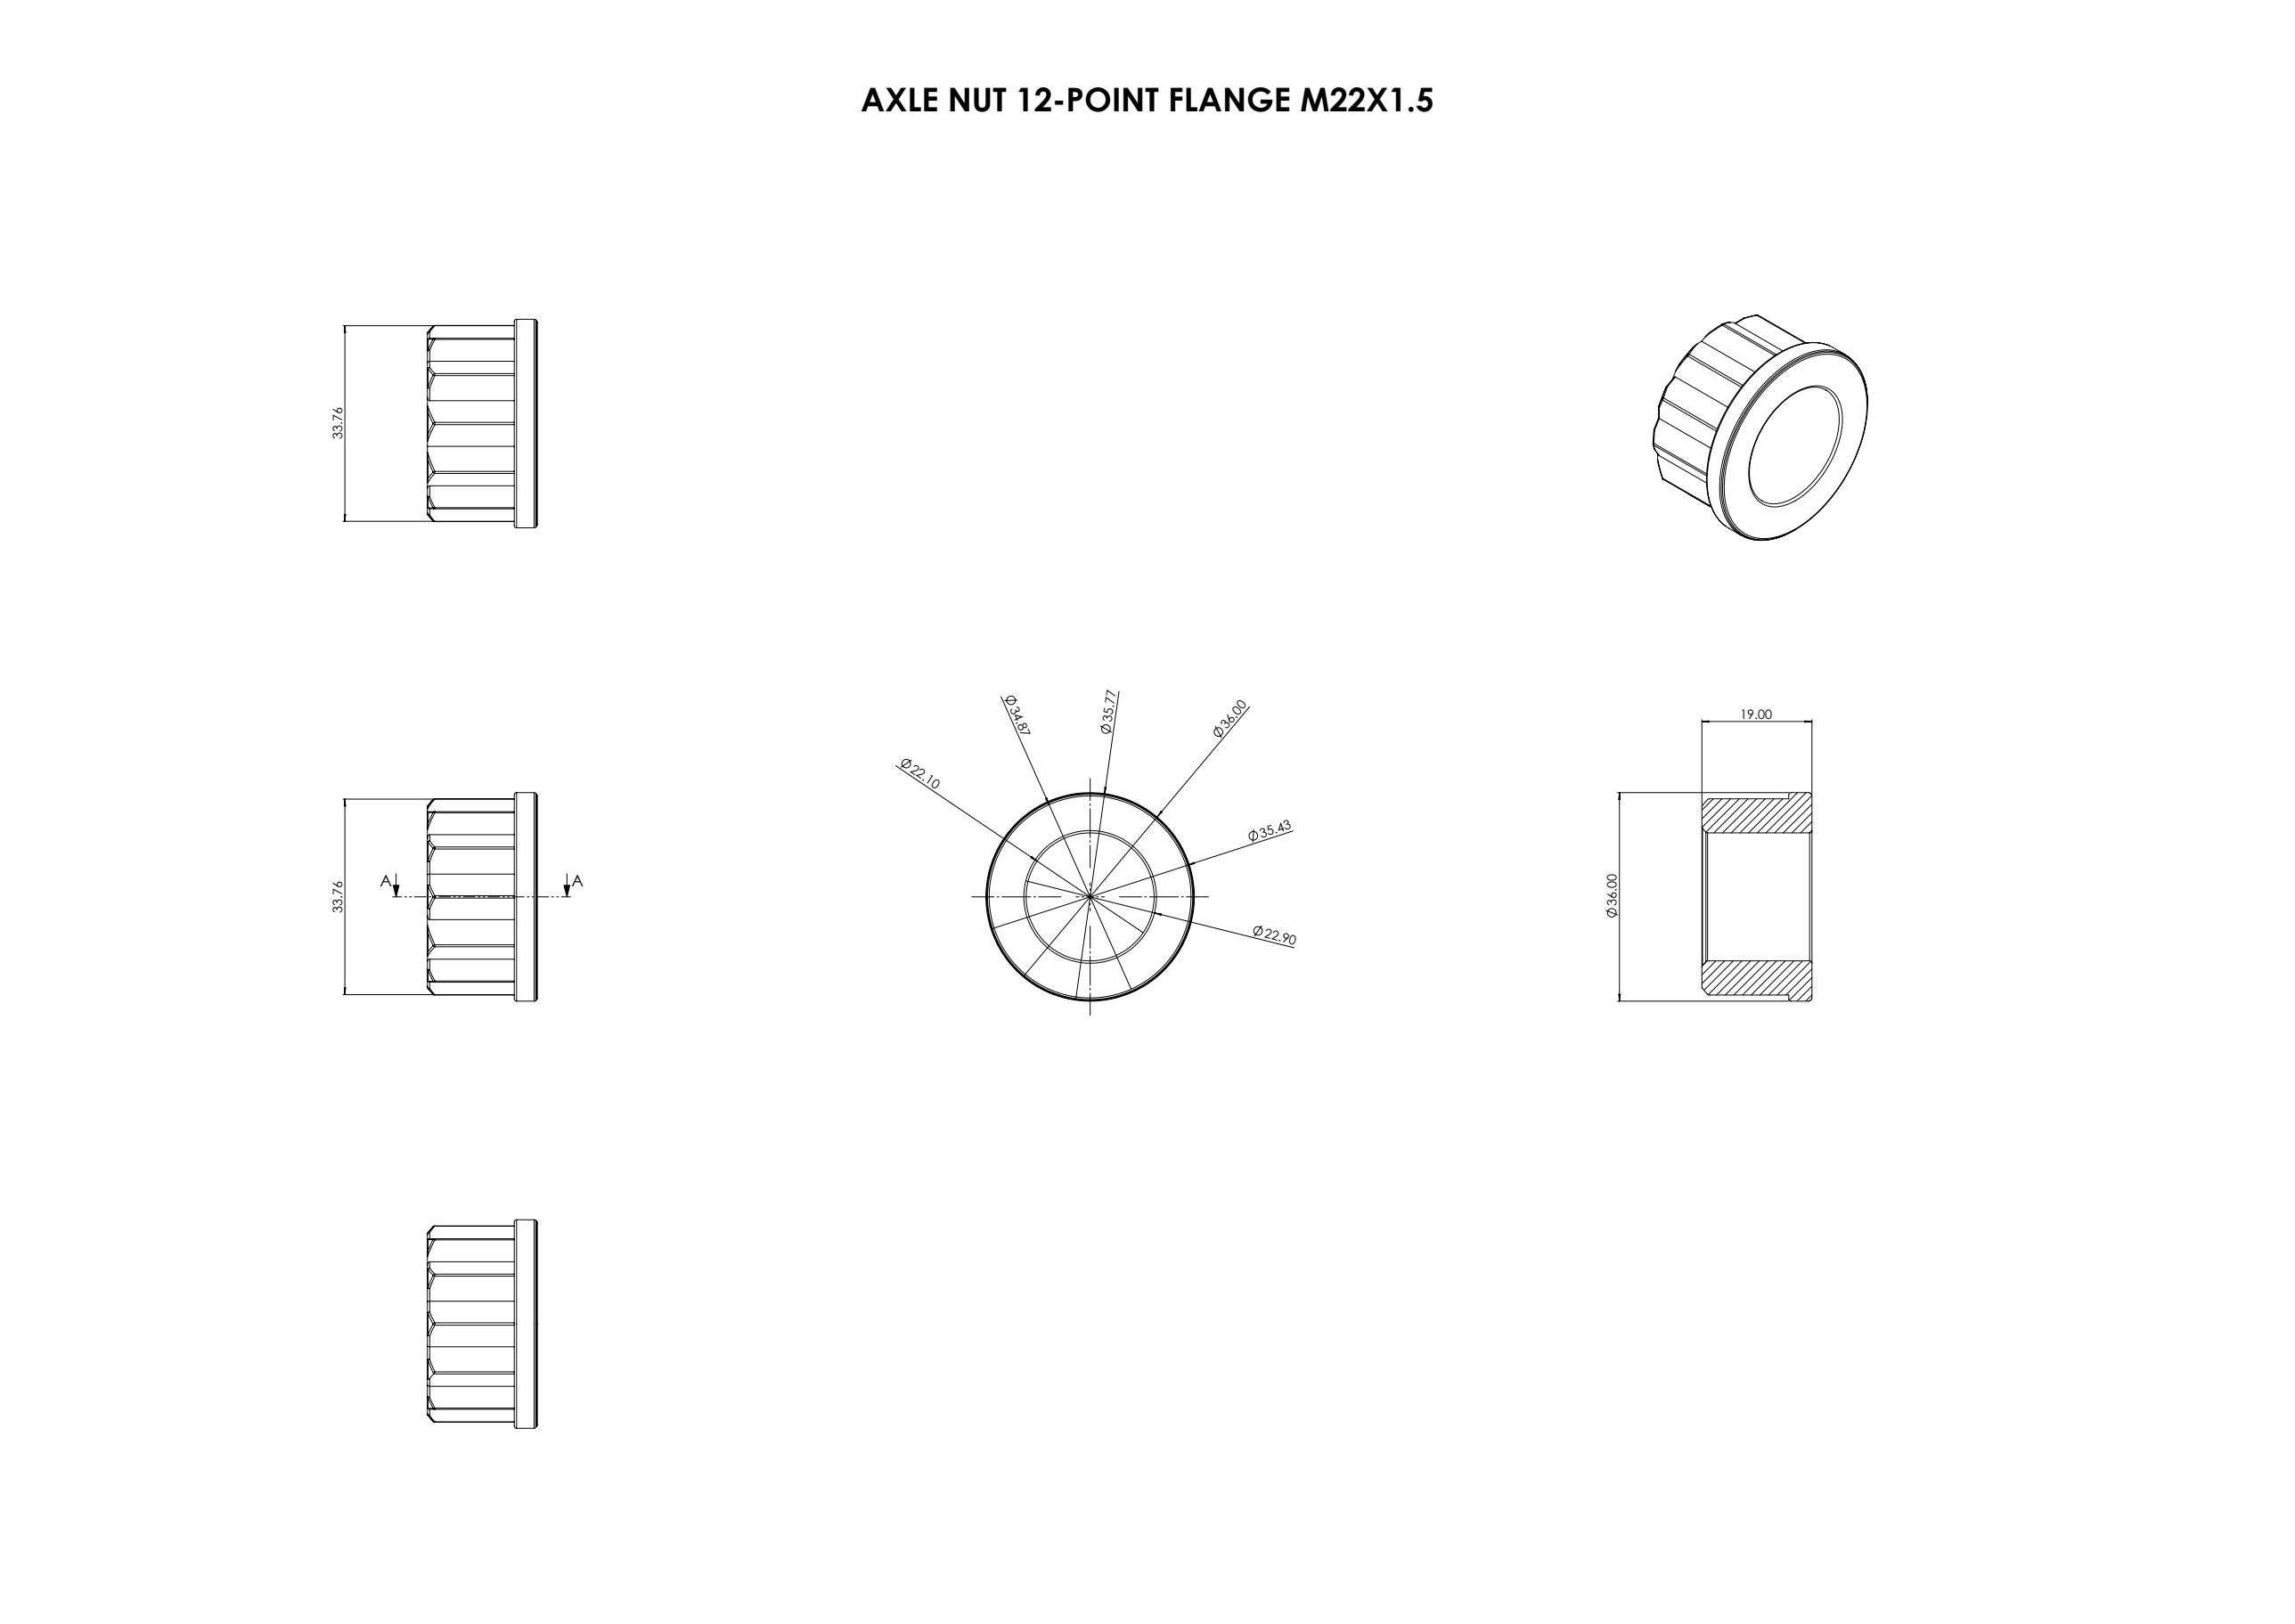
ISO-10303-21;
HEADER;
/* Generated by software containing ST-Developer
 * from STEP Tools, Inc. (www.steptools.com) 
 */

FILE_DESCRIPTION(
/* description */ (''),
/* implementation_level */ '2;1');

FILE_NAME(
/* name */ '03_Axle_Nut_12-Point_Flange_M22x1.5.step',
/* time_stamp */ '2026-10-11T12:57:03-07:00',
/* author */ (''),
/* organization */ (''),
/* preprocessor_version */ 'ST-DEVELOPER v20.2',
/* originating_system */ 'Autodesk Translation Framework v15.15.0.0',
/* authorisation */ '');

FILE_SCHEMA (('AUTOMOTIVE_DESIGN { 1 0 10303 214 3 1 1 }'));
ENDSEC;

DATA;
#10=MECHANICAL_DESIGN_GEOMETRIC_PRESENTATION_REPRESENTATION('',(#258),#90374);
#211=ELLIPSE('',#43033,0.776351396846868,0.4);
#212=ELLIPSE('',#43090,0.415109817788689,0.4);
#213=ELLIPSE('',#43102,0.776351396846869,0.4);
#214=ELLIPSE('',#43130,0.415109817788689,0.4);
#215=ELLIPSE('',#43133,0.41510981778869,0.4);
#216=ELLIPSE('',#43137,0.415109817788689,0.4);
#217=ELLIPSE('',#43157,0.41510981778869,0.4);
#218=ELLIPSE('',#43169,0.415109817788689,0.4);
#219=ELLIPSE('',#43208,0.776351396846868,0.4);
#220=ELLIPSE('',#43220,0.415109817788689,0.4);
#221=ELLIPSE('',#43243,0.776351396846868,0.4);
#224=SHAPE_REPRESENTATION_RELATIONSHIP('SRR','None',#90443,#241);
#241=ADVANCED_BREP_SHAPE_REPRESENTATION('',(#275),#90359);
#258=STYLED_ITEM('',(#90694),#275);
#275=MANIFOLD_SOLID_BREP('Body1',#40347);
#505=SPHERICAL_SURFACE('',#43027,0.4);
#506=SPHERICAL_SURFACE('',#43059,0.4);
#507=SPHERICAL_SURFACE('',#43061,0.4);
#508=SPHERICAL_SURFACE('',#43083,0.4);
#509=SPHERICAL_SURFACE('',#43093,0.4);
#510=SPHERICAL_SURFACE('',#43095,0.4);
#511=SPHERICAL_SURFACE('',#43105,0.4);
#512=SPHERICAL_SURFACE('',#43109,0.4);
#513=SPHERICAL_SURFACE('',#43121,0.4);
#514=SPHERICAL_SURFACE('',#43142,0.4);
#515=SPHERICAL_SURFACE('',#43145,0.4);
#516=SPHERICAL_SURFACE('',#43147,0.4);
#517=SPHERICAL_SURFACE('',#43160,0.4);
#518=SPHERICAL_SURFACE('',#43172,0.399999999999999);
#519=SPHERICAL_SURFACE('',#43181,0.4);
#520=SPHERICAL_SURFACE('',#43183,0.4);
#521=SPHERICAL_SURFACE('',#43185,0.4);
#522=SPHERICAL_SURFACE('',#43187,0.4);
#523=SPHERICAL_SURFACE('',#43189,0.4);
#524=SPHERICAL_SURFACE('',#43202,0.4);
#525=SPHERICAL_SURFACE('',#43210,0.4);
#526=SPHERICAL_SURFACE('',#43225,0.4);
#527=SPHERICAL_SURFACE('',#43228,0.4);
#528=SPHERICAL_SURFACE('',#43231,0.4);
#529=SPHERICAL_SURFACE('',#43237,0.4);
#530=SPHERICAL_SURFACE('',#43244,0.4);
#531=SPHERICAL_SURFACE('',#43258,0.4);
#532=SPHERICAL_SURFACE('',#43261,0.4);
#673=CONICAL_SURFACE('',#43008,17.8,0.785398163397448);
#674=CONICAL_SURFACE('',#43050,11.55,0.83798122500839);
#675=CONICAL_SURFACE('',#43065,16.55,0.840896668643165);
#676=CONICAL_SURFACE('',#43114,16.55,0.840896668643165);
#677=CONICAL_SURFACE('',#43124,16.55,0.840896668643165);
#678=CONICAL_SURFACE('',#43127,16.55,0.840896668643165);
#679=CONICAL_SURFACE('',#43152,16.55,0.840896668643165);
#680=CONICAL_SURFACE('',#43191,16.55,0.840896668643165);
#681=CONICAL_SURFACE('',#43194,16.55,0.840896668643165);
#682=CONICAL_SURFACE('',#43209,16.55,0.840896668643165);
#683=CONICAL_SURFACE('',#43229,16.55,0.840896668643165);
#684=CONICAL_SURFACE('',#43262,16.55,0.840896668643165);
#685=CONICAL_SURFACE('',#43267,16.55,0.840896668643165);
#686=CONICAL_SURFACE('',#43271,16.55,0.840896668643165);
#955=TOROIDAL_SURFACE('',#42999,17.6,0.4);
#956=TOROIDAL_SURFACE('',#43011,17.6,0.4);
#957=TOROIDAL_SURFACE('',#43034,17.4343145750508,0.4);
#958=TOROIDAL_SURFACE('',#43039,11.45,0.4);
#959=TOROIDAL_SURFACE('',#43046,11.45,0.4);
#960=TOROIDAL_SURFACE('',#43067,15.5589388807538,0.4);
#961=TOROIDAL_SURFACE('',#43111,15.5589388807538,0.4);
#962=TOROIDAL_SURFACE('',#43126,15.5589388807538,0.4);
#963=TOROIDAL_SURFACE('',#43131,15.5589388807538,0.4);
#964=TOROIDAL_SURFACE('',#43149,15.5589388807538,0.4);
#965=TOROIDAL_SURFACE('',#43193,15.5589388807538,0.4);
#966=TOROIDAL_SURFACE('',#43196,15.5589388807538,0.4);
#967=TOROIDAL_SURFACE('',#43203,12.0923832909811,0.4);
#968=TOROIDAL_SURFACE('',#43205,15.5589388807538,0.4);
#969=TOROIDAL_SURFACE('',#43221,15.5589388807538,0.4);
#970=TOROIDAL_SURFACE('',#43254,15.5589388807538,0.4);
#971=TOROIDAL_SURFACE('',#43264,15.5589388807538,0.4);
#972=TOROIDAL_SURFACE('',#43268,15.5589388807538,0.4);
#1049=FACE_BOUND('',#5817,.T.);
#1050=FACE_BOUND('',#5825,.T.);
#1051=FACE_BOUND('',#5840,.T.);
#1302=PLANE('',#43014);
#1303=PLANE('',#43032);
#1304=PLANE('',#43037);
#1305=PLANE('',#43063);
#1306=PLANE('',#43070);
#1307=PLANE('',#43097);
#1308=PLANE('',#43099);
#1309=PLANE('',#43116);
#1310=PLANE('',#43123);
#1311=PLANE('',#43134);
#1312=PLANE('',#43148);
#1313=PLANE('',#43190);
#1314=PLANE('',#43197);
#1315=PLANE('',#43198);
#1316=PLANE('',#43199);
#1317=PLANE('',#43207);
#1318=PLANE('',#43215);
#1319=PLANE('',#43230);
#1320=PLANE('',#43236);
#1321=PLANE('',#43242);
#1322=PLANE('',#43249);
#1323=PLANE('',#43263);
#1324=PLANE('',#43266);
#1325=PLANE('',#43270);
#1326=PLANE('',#43272);
#1327=PLANE('',#43273);
#1328=PLANE('',#43274);
#1830=(
BOUNDED_CURVE()
B_SPLINE_CURVE(2,(#77759,#77760,#77761),.UNSPECIFIED.,.F.,.F.)
B_SPLINE_CURVE_WITH_KNOTS((3,3),(0.123046239516649,0.293199132396535),
 .UNSPECIFIED.)
CURVE()
GEOMETRIC_REPRESENTATION_ITEM()
RATIONAL_B_SPLINE_CURVE((1.00286885652603,1.0040332208536,1.00293190037169))
REPRESENTATION_ITEM('')
);
#2083=B_SPLINE_SURFACE_WITH_KNOTS('',3,3,((#77247,#77248,#77249,#77250),
(#77251,#77252,#77253,#77254),(#77255,#77256,#77257,#77258),(#77259,#77260,
#77261,#77262)),.UNSPECIFIED.,.F.,.F.,.F.,(4,4),(4,4),(0.,1.),(0.238859576382585,
0.597949259053295),.UNSPECIFIED.);
#2084=B_SPLINE_SURFACE_WITH_KNOTS('',3,3,((#77282,#77283,#77284,#77285),
(#77286,#77287,#77288,#77289),(#77290,#77291,#77292,#77293),(#77294,#77295,
#77296,#77297)),.UNSPECIFIED.,.F.,.F.,.F.,(4,4),(4,4),(0.,1.),(0.161384884357676,
0.520475215840057),.UNSPECIFIED.);
#2085=B_SPLINE_SURFACE_WITH_KNOTS('',3,3,((#77359,#77360,#77361,#77362),
(#77363,#77364,#77365,#77366),(#77367,#77368,#77369,#77370),(#77371,#77372,
#77373,#77374)),.UNSPECIFIED.,.F.,.F.,.F.,(4,4),(4,4),(0.,1.),(0.,0.231241687907805),
 .UNSPECIFIED.);
#2086=B_SPLINE_SURFACE_WITH_KNOTS('',3,3,((#77406,#77407,#77408,#77409),
(#77410,#77411,#77412,#77413),(#77414,#77415,#77416,#77417),(#77418,#77419,
#77420,#77421)),.UNSPECIFIED.,.F.,.F.,.F.,(4,4),(4,4),(0.,1.),(0.232923065268537,
0.464164679032266),.UNSPECIFIED.);
#2087=B_SPLINE_SURFACE_WITH_KNOTS('',3,3,((#77539,#77540,#77541,#77542),
(#77543,#77544,#77545,#77546),(#77547,#77548,#77549,#77550),(#77551,#77552,
#77553,#77554)),.UNSPECIFIED.,.F.,.F.,.F.,(4,4),(4,4),(0.,1.),(0.,0.23124168790661),
 .UNSPECIFIED.);
#2088=B_SPLINE_SURFACE_WITH_KNOTS('',3,3,((#77572,#77573,#77574,#77575),
(#77576,#77577,#77578,#77579),(#77580,#77581,#77582,#77583),(#77584,#77585,
#77586,#77587)),.UNSPECIFIED.,.F.,.F.,.F.,(4,4),(4,4),(0.,1.),(0.,0.2312416879078),
 .UNSPECIFIED.);
#2089=B_SPLINE_SURFACE_WITH_KNOTS('',3,3,((#77617,#77618,#77619,#77620),
(#77621,#77622,#77623,#77624),(#77625,#77626,#77627,#77628),(#77629,#77630,
#77631,#77632)),.UNSPECIFIED.,.F.,.F.,.F.,(4,4),(4,4),(0.,1.),(0.,0.231241687907749),
 .UNSPECIFIED.);
#2090=B_SPLINE_SURFACE_WITH_KNOTS('',3,3,((#77664,#77665,#77666,#77667),
(#77668,#77669,#77670,#77671),(#77672,#77673,#77674,#77675),(#77676,#77677,
#77678,#77679)),.UNSPECIFIED.,.F.,.F.,.F.,(4,4),(4,4),(0.,1.),(0.,0.231241350797188),
 .UNSPECIFIED.);
#2091=B_SPLINE_SURFACE_WITH_KNOTS('',3,3,((#77725,#77726,#77727,#77728),
(#77729,#77730,#77731,#77732),(#77733,#77734,#77735,#77736),(#77737,#77738,
#77739,#77740)),.UNSPECIFIED.,.F.,.F.,.F.,(4,4),(4,4),(0.,1.),(0.,0.252215655062094),
 .UNSPECIFIED.);
#2092=B_SPLINE_SURFACE_WITH_KNOTS('',3,3,((#77807,#77808,#77809,#77810),
(#77811,#77812,#77813,#77814),(#77815,#77816,#77817,#77818),(#77819,#77820,
#77821,#77822)),.UNSPECIFIED.,.F.,.F.,.F.,(4,4),(4,4),(0.,1.),(0.,0.231241687907802),
 .UNSPECIFIED.);
#2093=B_SPLINE_SURFACE_WITH_KNOTS('',3,3,((#77857,#77858,#77859,#77860),
(#77861,#77862,#77863,#77864),(#77865,#77866,#77867,#77868),(#77869,#77870,
#77871,#77872)),.UNSPECIFIED.,.F.,.F.,.F.,(4,4),(4,4),(0.,1.),(0.,0.231241586165377),
 .UNSPECIFIED.);
#2094=B_SPLINE_SURFACE_WITH_KNOTS('',3,3,((#77898,#77899,#77900,#77901),
(#77902,#77903,#77904,#77905),(#77906,#77907,#77908,#77909),(#77910,#77911,
#77912,#77913)),.UNSPECIFIED.,.F.,.F.,.F.,(4,4),(4,4),(0.,1.),(0.,0.23124114363781),
 .UNSPECIFIED.);
#2095=B_SPLINE_SURFACE_WITH_KNOTS('',3,3,((#77925,#77926,#77927,#77928),
(#77929,#77930,#77931,#77932),(#77933,#77934,#77935,#77936),(#77937,#77938,
#77939,#77940)),.UNSPECIFIED.,.F.,.F.,.F.,(4,4),(4,4),(0.,1.),(0.228586915697378,
0.459828059335187),.UNSPECIFIED.);
#2096=B_SPLINE_SURFACE_WITH_KNOTS('',3,3,((#77970,#77971,#77972,#77973),
(#77974,#77975,#77976,#77977),(#77978,#77979,#77980,#77981),(#77982,#77983,
#77984,#77985)),.UNSPECIFIED.,.F.,.F.,.F.,(4,4),(4,4),(0.,1.),(0.,0.231241350797186),
 .UNSPECIFIED.);
#2097=B_SPLINE_SURFACE_WITH_KNOTS('',3,3,((#77997,#77998,#77999,#78000),
(#78001,#78002,#78003,#78004),(#78005,#78006,#78007,#78008),(#78009,#78010,
#78011,#78012)),.UNSPECIFIED.,.F.,.F.,.F.,(4,4),(4,4),(0.,1.),(0.215800706400213,
0.447042292565588),.UNSPECIFIED.);
#2098=B_SPLINE_SURFACE_WITH_KNOTS('',3,3,((#78076,#78077,#78078,#78079),
(#78080,#78081,#78082,#78083),(#78084,#78085,#78086,#78087),(#78088,#78089,
#78090,#78091)),.UNSPECIFIED.,.F.,.F.,.F.,(4,4),(4,4),(0.,1.),(0.228585906851782,
0.459827831361922),.UNSPECIFIED.);
#2099=B_SPLINE_SURFACE_WITH_KNOTS('',3,3,((#78098,#78099,#78100,#78101),
(#78102,#78103,#78104,#78105),(#78106,#78107,#78108,#78109),(#78110,#78111,
#78112,#78113)),.UNSPECIFIED.,.F.,.F.,.F.,(4,4),(4,4),(0.,1.),(0.289233280455309,
0.520475100360999),.UNSPECIFIED.);
#2100=B_SPLINE_SURFACE_WITH_KNOTS('',3,3,((#78157,#78158,#78159,#78160),
(#78161,#78162,#78163,#78164),(#78165,#78166,#78167,#78168),(#78169,#78170,
#78171,#78172)),.UNSPECIFIED.,.F.,.F.,.F.,(4,4),(4,4),(0.,1.),(0.228585906851781,
0.587676103485633),.UNSPECIFIED.);
#2101=B_SPLINE_SURFACE_WITH_KNOTS('',3,3,((#78184,#78185,#78186,#78187),
(#78188,#78189,#78190,#78191),(#78192,#78193,#78194,#78195),(#78196,#78197,
#78198,#78199)),.UNSPECIFIED.,.F.,.F.,.F.,(4,4),(4,4),(0.,1.),(0.157372832782455,
0.516463029416307),.UNSPECIFIED.);
#2102=B_SPLINE_SURFACE_WITH_KNOTS('',3,3,((#78233,#78234,#78235,#78236),
(#78237,#78238,#78239,#78240),(#78241,#78242,#78243,#78244),(#78245,#78246,
#78247,#78248)),.UNSPECIFIED.,.F.,.F.,.F.,(4,4),(4,4),(0.,1.),(0.238859576382585,
0.597949259053296),.UNSPECIFIED.);
#2103=B_SPLINE_SURFACE_WITH_KNOTS('',3,3,((#78260,#78261,#78262,#78263),
(#78264,#78265,#78266,#78267),(#78268,#78269,#78270,#78271),(#78272,#78273,
#78274,#78275)),.UNSPECIFIED.,.F.,.F.,.F.,(4,4),(4,4),(0.,1.),(0.14489400298759,
0.503986701734181),.UNSPECIFIED.);
#2104=B_SPLINE_SURFACE_WITH_KNOTS('',3,3,((#78308,#78309,#78310,#78311),
(#78312,#78313,#78314,#78315),(#78316,#78317,#78318,#78319),(#78320,#78321,
#78322,#78323)),.UNSPECIFIED.,.F.,.F.,.F.,(4,4),(4,4),(0.,1.),(0.232923065268538,
0.464164679032267),.UNSPECIFIED.);
#2105=B_SPLINE_SURFACE_WITH_KNOTS('',3,3,((#78330,#78331,#78332,#78333),
(#78334,#78335,#78336,#78337),(#78338,#78339,#78340,#78341),(#78342,#78343,
#78344,#78345)),.UNSPECIFIED.,.F.,.F.,.F.,(4,4),(4,4),(0.,1.),(0.27134084970268,
0.502582702411899),.UNSPECIFIED.);
#3406=FACE_OUTER_BOUND('',#5812,.T.);
#3407=FACE_OUTER_BOUND('',#5813,.T.);
#3408=FACE_OUTER_BOUND('',#5814,.T.);
#3409=FACE_OUTER_BOUND('',#5815,.T.);
#3410=FACE_OUTER_BOUND('',#5816,.T.);
#3411=FACE_OUTER_BOUND('',#5818,.T.);
#3412=FACE_OUTER_BOUND('',#5819,.T.);
#3413=FACE_OUTER_BOUND('',#5820,.T.);
#3414=FACE_OUTER_BOUND('',#5821,.T.);
#3415=FACE_OUTER_BOUND('',#5822,.T.);
#3416=FACE_OUTER_BOUND('',#5823,.T.);
#3417=FACE_OUTER_BOUND('',#5824,.T.);
#3418=FACE_OUTER_BOUND('',#5826,.T.);
#3419=FACE_OUTER_BOUND('',#5827,.T.);
#3420=FACE_OUTER_BOUND('',#5828,.T.);
#3421=FACE_OUTER_BOUND('',#5829,.T.);
#3422=FACE_OUTER_BOUND('',#5830,.T.);
#3423=FACE_OUTER_BOUND('',#5831,.T.);
#3424=FACE_OUTER_BOUND('',#5832,.T.);
#3425=FACE_OUTER_BOUND('',#5833,.T.);
#3426=FACE_OUTER_BOUND('',#5834,.T.);
#3427=FACE_OUTER_BOUND('',#5835,.T.);
#3428=FACE_OUTER_BOUND('',#5836,.T.);
#3429=FACE_OUTER_BOUND('',#5837,.T.);
#3430=FACE_OUTER_BOUND('',#5838,.T.);
#3431=FACE_OUTER_BOUND('',#5839,.T.);
#3432=FACE_OUTER_BOUND('',#5841,.T.);
#3433=FACE_OUTER_BOUND('',#5842,.T.);
#3434=FACE_OUTER_BOUND('',#5843,.T.);
#3435=FACE_OUTER_BOUND('',#5844,.T.);
#3436=FACE_OUTER_BOUND('',#5845,.T.);
#3437=FACE_OUTER_BOUND('',#5846,.T.);
#3438=FACE_OUTER_BOUND('',#5847,.T.);
#3439=FACE_OUTER_BOUND('',#5848,.T.);
#3440=FACE_OUTER_BOUND('',#5849,.T.);
#3441=FACE_OUTER_BOUND('',#5850,.T.);
#3442=FACE_OUTER_BOUND('',#5851,.T.);
#3443=FACE_OUTER_BOUND('',#5852,.T.);
#3444=FACE_OUTER_BOUND('',#5853,.T.);
#3445=FACE_OUTER_BOUND('',#5854,.T.);
#3446=FACE_OUTER_BOUND('',#5855,.T.);
#3447=FACE_OUTER_BOUND('',#5856,.T.);
#3448=FACE_OUTER_BOUND('',#5857,.T.);
#3449=FACE_OUTER_BOUND('',#5858,.T.);
#3450=FACE_OUTER_BOUND('',#5859,.T.);
#3451=FACE_OUTER_BOUND('',#5860,.T.);
#3452=FACE_OUTER_BOUND('',#5861,.T.);
#3453=FACE_OUTER_BOUND('',#5862,.T.);
#3454=FACE_OUTER_BOUND('',#5863,.T.);
#3455=FACE_OUTER_BOUND('',#5864,.T.);
#3456=FACE_OUTER_BOUND('',#5865,.T.);
#3457=FACE_OUTER_BOUND('',#5866,.T.);
#3458=FACE_OUTER_BOUND('',#5867,.T.);
#3459=FACE_OUTER_BOUND('',#5868,.T.);
#3460=FACE_OUTER_BOUND('',#5869,.T.);
#3461=FACE_OUTER_BOUND('',#5870,.T.);
#3462=FACE_OUTER_BOUND('',#5871,.T.);
#3463=FACE_OUTER_BOUND('',#5872,.T.);
#3464=FACE_OUTER_BOUND('',#5873,.T.);
#3465=FACE_OUTER_BOUND('',#5874,.T.);
#3466=FACE_OUTER_BOUND('',#5875,.T.);
#3467=FACE_OUTER_BOUND('',#5876,.T.);
#3468=FACE_OUTER_BOUND('',#5877,.T.);
#3469=FACE_OUTER_BOUND('',#5878,.T.);
#3470=FACE_OUTER_BOUND('',#5879,.T.);
#3471=FACE_OUTER_BOUND('',#5880,.T.);
#3472=FACE_OUTER_BOUND('',#5881,.T.);
#3473=FACE_OUTER_BOUND('',#5882,.T.);
#3474=FACE_OUTER_BOUND('',#5883,.T.);
#3475=FACE_OUTER_BOUND('',#5884,.T.);
#3476=FACE_OUTER_BOUND('',#5885,.T.);
#3477=FACE_OUTER_BOUND('',#5886,.T.);
#3478=FACE_OUTER_BOUND('',#5887,.T.);
#3479=FACE_OUTER_BOUND('',#5888,.T.);
#3480=FACE_OUTER_BOUND('',#5889,.T.);
#3481=FACE_OUTER_BOUND('',#5890,.T.);
#3482=FACE_OUTER_BOUND('',#5891,.T.);
#3483=FACE_OUTER_BOUND('',#5892,.T.);
#3484=FACE_OUTER_BOUND('',#5893,.T.);
#3485=FACE_OUTER_BOUND('',#5894,.T.);
#3486=FACE_OUTER_BOUND('',#5895,.T.);
#3487=FACE_OUTER_BOUND('',#5896,.T.);
#3488=FACE_OUTER_BOUND('',#5897,.T.);
#3489=FACE_OUTER_BOUND('',#5898,.T.);
#3490=FACE_OUTER_BOUND('',#5899,.T.);
#3491=FACE_OUTER_BOUND('',#5900,.T.);
#3492=FACE_OUTER_BOUND('',#5901,.T.);
#3493=FACE_OUTER_BOUND('',#5902,.T.);
#3494=FACE_OUTER_BOUND('',#5903,.T.);
#3495=FACE_OUTER_BOUND('',#5904,.T.);
#3496=FACE_OUTER_BOUND('',#5905,.T.);
#3497=FACE_OUTER_BOUND('',#5906,.T.);
#3498=FACE_OUTER_BOUND('',#5907,.T.);
#3499=FACE_OUTER_BOUND('',#5908,.T.);
#3500=FACE_OUTER_BOUND('',#5909,.T.);
#3501=FACE_OUTER_BOUND('',#5910,.T.);
#3502=FACE_OUTER_BOUND('',#5911,.T.);
#3503=FACE_OUTER_BOUND('',#5912,.T.);
#3504=FACE_OUTER_BOUND('',#5913,.T.);
#3505=FACE_OUTER_BOUND('',#5914,.T.);
#3506=FACE_OUTER_BOUND('',#5915,.T.);
#3507=FACE_OUTER_BOUND('',#5916,.T.);
#3508=FACE_OUTER_BOUND('',#5917,.T.);
#3509=FACE_OUTER_BOUND('',#5918,.T.);
#3510=FACE_OUTER_BOUND('',#5919,.T.);
#3511=FACE_OUTER_BOUND('',#5920,.T.);
#3512=FACE_OUTER_BOUND('',#5921,.T.);
#3513=FACE_OUTER_BOUND('',#5922,.T.);
#3514=FACE_OUTER_BOUND('',#5923,.T.);
#3515=FACE_OUTER_BOUND('',#5924,.T.);
#3516=FACE_OUTER_BOUND('',#5925,.T.);
#3517=FACE_OUTER_BOUND('',#5926,.T.);
#3518=FACE_OUTER_BOUND('',#5927,.T.);
#3519=FACE_OUTER_BOUND('',#5928,.T.);
#3520=FACE_OUTER_BOUND('',#5929,.T.);
#3521=FACE_OUTER_BOUND('',#5930,.T.);
#3522=FACE_OUTER_BOUND('',#5931,.T.);
#3523=FACE_OUTER_BOUND('',#5932,.T.);
#3524=FACE_OUTER_BOUND('',#5933,.T.);
#3525=FACE_OUTER_BOUND('',#5934,.T.);
#3526=FACE_OUTER_BOUND('',#5935,.T.);
#3527=FACE_OUTER_BOUND('',#5936,.T.);
#3528=FACE_OUTER_BOUND('',#5937,.T.);
#3529=FACE_OUTER_BOUND('',#5938,.T.);
#3530=FACE_OUTER_BOUND('',#5939,.T.);
#3531=FACE_OUTER_BOUND('',#5940,.T.);
#3532=FACE_OUTER_BOUND('',#5941,.T.);
#3533=FACE_OUTER_BOUND('',#5942,.T.);
#3534=FACE_OUTER_BOUND('',#5943,.T.);
#3535=FACE_OUTER_BOUND('',#5944,.T.);
#3536=FACE_OUTER_BOUND('',#5945,.T.);
#3537=FACE_OUTER_BOUND('',#5946,.T.);
#3538=FACE_OUTER_BOUND('',#5947,.T.);
#3539=FACE_OUTER_BOUND('',#5948,.T.);
#3540=FACE_OUTER_BOUND('',#5949,.T.);
#3541=FACE_OUTER_BOUND('',#5950,.T.);
#3542=FACE_OUTER_BOUND('',#5951,.T.);
#3543=FACE_OUTER_BOUND('',#5952,.T.);
#3544=FACE_OUTER_BOUND('',#5953,.T.);
#3545=FACE_OUTER_BOUND('',#5954,.T.);
#3546=FACE_OUTER_BOUND('',#5955,.T.);
#3547=FACE_OUTER_BOUND('',#5956,.T.);
#5812=EDGE_LOOP('',(#31161,#31162,#31163,#31164,#31165,#31166));
#5813=EDGE_LOOP('',(#31167,#31168,#31169,#31170,#31171,#31172));
#5814=EDGE_LOOP('',(#31173,#31174,#31175,#31176,#31177,#31178));
#5815=EDGE_LOOP('',(#31179,#31180,#31181,#31182,#31183));
#5816=EDGE_LOOP('',(#31184));
#5817=EDGE_LOOP('',(#31185,#31186,#31187,#31188,#31189,#31190,#31191,#31192,
#31193,#31194,#31195,#31196,#31197,#31198,#31199,#31200,#31201,#31202,#31203,
#31204,#31205,#31206,#31207,#31208,#31209,#31210,#31211,#31212,#31213,#31214,
#31215,#31216,#31217,#31218,#31219,#31220));
#5818=EDGE_LOOP('',(#31221,#31222,#31223));
#5819=EDGE_LOOP('',(#31224,#31225,#31226,#31227));
#5820=EDGE_LOOP('',(#31228,#31229,#31230,#31231,#31232,#31233));
#5821=EDGE_LOOP('',(#31234,#31235,#31236,#31237,#31238));
#5822=EDGE_LOOP('',(#31239,#31240,#31241,#31242,#31243));
#5823=EDGE_LOOP('',(#31244,#31245,#31246,#31247,#31248));
#5824=EDGE_LOOP('',(#31249));
#5825=EDGE_LOOP('',(#31250));
#5826=EDGE_LOOP('',(#31251,#31252,#31253,#31254,#31255));
#5827=EDGE_LOOP('',(#31256,#31257,#31258,#31259,#31260,#31261));
#5828=EDGE_LOOP('',(#31262,#31263,#31264,#31265,#31266,#31267));
#5829=EDGE_LOOP('',(#31268,#31269,#31270,#31271,#31272,#31273));
#5830=EDGE_LOOP('',(#31274,#31275,#31276,#31277));
#5831=EDGE_LOOP('',(#31278,#31279,#31280,#31281));
#5832=EDGE_LOOP('',(#31282,#31283,#31284,#31285));
#5833=EDGE_LOOP('',(#31286,#31287,#31288));
#5834=EDGE_LOOP('',(#31289,#31290,#31291));
#5835=EDGE_LOOP('',(#31292,#31293,#31294,#31295,#31296));
#5836=EDGE_LOOP('',(#31297,#31298,#31299,#31300));
#5837=EDGE_LOOP('',(#31301,#31302,#31303));
#5838=EDGE_LOOP('',(#31304,#31305,#31306,#31307));
#5839=EDGE_LOOP('',(#31308,#31309,#31310,#31311,#31312,#31313,#31314,#31315,
#31316,#31317,#31318,#31319,#31320,#31321,#31322,#31323,#31324,#31325,#31326,
#31327,#31328,#31329,#31330,#31331,#31332,#31333,#31334,#31335,#31336,#31337,
#31338,#31339,#31340,#31341,#31342,#31343,#31344,#31345,#31346,#31347,#31348,
#31349));
#5840=EDGE_LOOP('',(#31350));
#5841=EDGE_LOOP('',(#31351,#31352,#31353));
#5842=EDGE_LOOP('',(#31354,#31355,#31356,#31357));
#5843=EDGE_LOOP('',(#31358,#31359,#31360,#31361));
#5844=EDGE_LOOP('',(#31362,#31363,#31364,#31365));
#5845=EDGE_LOOP('',(#31366,#31367,#31368));
#5846=EDGE_LOOP('',(#31369,#31370,#31371));
#5847=EDGE_LOOP('',(#31372,#31373,#31374,#31375,#31376));
#5848=EDGE_LOOP('',(#31377,#31378,#31379,#31380));
#5849=EDGE_LOOP('',(#31381,#31382,#31383,#31384,#31385));
#5850=EDGE_LOOP('',(#31386,#31387,#31388,#31389));
#5851=EDGE_LOOP('',(#31390,#31391,#31392,#31393));
#5852=EDGE_LOOP('',(#31394,#31395,#31396));
#5853=EDGE_LOOP('',(#31397,#31398,#31399,#31400));
#5854=EDGE_LOOP('',(#31401,#31402,#31403));
#5855=EDGE_LOOP('',(#31404,#31405,#31406,#31407));
#5856=EDGE_LOOP('',(#31408,#31409,#31410));
#5857=EDGE_LOOP('',(#31411,#31412,#31413,#31414));
#5858=EDGE_LOOP('',(#31415,#31416,#31417,#31418,#31419));
#5859=EDGE_LOOP('',(#31420,#31421,#31422,#31423,#31424));
#5860=EDGE_LOOP('',(#31425,#31426,#31427,#31428));
#5861=EDGE_LOOP('',(#31429,#31430,#31431,#31432));
#5862=EDGE_LOOP('',(#31433,#31434,#31435));
#5863=EDGE_LOOP('',(#31436,#31437,#31438,#31439,#31440));
#5864=EDGE_LOOP('',(#31441,#31442,#31443,#31444,#31445));
#5865=EDGE_LOOP('',(#31446,#31447,#31448,#31449));
#5866=EDGE_LOOP('',(#31450,#31451,#31452));
#5867=EDGE_LOOP('',(#31453,#31454,#31455,#31456));
#5868=EDGE_LOOP('',(#31457,#31458,#31459,#31460));
#5869=EDGE_LOOP('',(#31461,#31462,#31463,#31464,#31465));
#5870=EDGE_LOOP('',(#31466,#31467,#31468,#31469,#31470));
#5871=EDGE_LOOP('',(#31471,#31472,#31473,#31474));
#5872=EDGE_LOOP('',(#31475,#31476,#31477,#31478));
#5873=EDGE_LOOP('',(#31479,#31480,#31481,#31482));
#5874=EDGE_LOOP('',(#31483,#31484,#31485));
#5875=EDGE_LOOP('',(#31486,#31487,#31488));
#5876=EDGE_LOOP('',(#31489,#31490,#31491));
#5877=EDGE_LOOP('',(#31492,#31493,#31494,#31495,#31496));
#5878=EDGE_LOOP('',(#31497,#31498,#31499,#31500));
#5879=EDGE_LOOP('',(#31501,#31502,#31503));
#5880=EDGE_LOOP('',(#31504,#31505,#31506,#31507));
#5881=EDGE_LOOP('',(#31508,#31509,#31510,#31511));
#5882=EDGE_LOOP('',(#31512,#31513,#31514,#31515));
#5883=EDGE_LOOP('',(#31516,#31517,#31518,#31519));
#5884=EDGE_LOOP('',(#31520,#31521,#31522));
#5885=EDGE_LOOP('',(#31523,#31524,#31525,#31526));
#5886=EDGE_LOOP('',(#31527,#31528,#31529,#31530));
#5887=EDGE_LOOP('',(#31531,#31532,#31533,#31534));
#5888=EDGE_LOOP('',(#31535,#31536,#31537,#31538));
#5889=EDGE_LOOP('',(#31539,#31540,#31541,#31542));
#5890=EDGE_LOOP('',(#31543,#31544,#31545));
#5891=EDGE_LOOP('',(#31546,#31547,#31548,#31549));
#5892=EDGE_LOOP('',(#31550,#31551,#31552,#31553));
#5893=EDGE_LOOP('',(#31554,#31555,#31556,#31557));
#5894=EDGE_LOOP('',(#31558,#31559,#31560,#31561));
#5895=EDGE_LOOP('',(#31562,#31563,#31564));
#5896=EDGE_LOOP('',(#31565,#31566,#31567));
#5897=EDGE_LOOP('',(#31568,#31569,#31570));
#5898=EDGE_LOOP('',(#31571,#31572,#31573));
#5899=EDGE_LOOP('',(#31574,#31575,#31576));
#5900=EDGE_LOOP('',(#31577,#31578,#31579,#31580,#31581));
#5901=EDGE_LOOP('',(#31582,#31583,#31584));
#5902=EDGE_LOOP('',(#31585,#31586,#31587,#31588));
#5903=EDGE_LOOP('',(#31589,#31590,#31591));
#5904=EDGE_LOOP('',(#31592,#31593,#31594,#31595));
#5905=EDGE_LOOP('',(#31596,#31597,#31598,#31599,#31600));
#5906=EDGE_LOOP('',(#31601,#31602,#31603,#31604,#31605));
#5907=EDGE_LOOP('',(#31606,#31607,#31608,#31609,#31610));
#5908=EDGE_LOOP('',(#31611,#31612,#31613,#31614));
#5909=EDGE_LOOP('',(#31615,#31616,#31617));
#5910=EDGE_LOOP('',(#31618,#31619,#31620,#31621,#31622));
#5911=EDGE_LOOP('',(#31623,#31624,#31625,#31626));
#5912=EDGE_LOOP('',(#31627,#31628,#31629,#31630,#31631,#31632));
#5913=EDGE_LOOP('',(#31633,#31634,#31635));
#5914=EDGE_LOOP('',(#31636,#31637,#31638));
#5915=EDGE_LOOP('',(#31639,#31640,#31641,#31642));
#5916=EDGE_LOOP('',(#31643,#31644,#31645,#31646,#31647));
#5917=EDGE_LOOP('',(#31648,#31649,#31650,#31651));
#5918=EDGE_LOOP('',(#31652,#31653,#31654,#31655));
#5919=EDGE_LOOP('',(#31656,#31657,#31658,#31659));
#5920=EDGE_LOOP('',(#31660,#31661,#31662,#31663));
#5921=EDGE_LOOP('',(#31664,#31665,#31666));
#5922=EDGE_LOOP('',(#31667,#31668,#31669,#31670));
#5923=EDGE_LOOP('',(#31671,#31672,#31673));
#5924=EDGE_LOOP('',(#31674,#31675,#31676));
#5925=EDGE_LOOP('',(#31677,#31678,#31679,#31680,#31681));
#5926=EDGE_LOOP('',(#31682,#31683,#31684));
#5927=EDGE_LOOP('',(#31685,#31686,#31687,#31688));
#5928=EDGE_LOOP('',(#31689,#31690,#31691,#31692,#31693));
#5929=EDGE_LOOP('',(#31694,#31695,#31696,#31697,#31698));
#5930=EDGE_LOOP('',(#31699,#31700,#31701,#31702,#31703));
#5931=EDGE_LOOP('',(#31704,#31705,#31706));
#5932=EDGE_LOOP('',(#31707,#31708,#31709,#31710));
#5933=EDGE_LOOP('',(#31711,#31712,#31713,#31714,#31715,#31716));
#5934=EDGE_LOOP('',(#31717,#31718,#31719,#31720,#31721));
#5935=EDGE_LOOP('',(#31722,#31723,#31724,#31725,#31726));
#5936=EDGE_LOOP('',(#31727,#31728,#31729));
#5937=EDGE_LOOP('',(#31730,#31731,#31732,#31733));
#5938=EDGE_LOOP('',(#31734,#31735,#31736,#31737,#31738));
#5939=EDGE_LOOP('',(#31739,#31740,#31741,#31742));
#5940=EDGE_LOOP('',(#31743,#31744,#31745,#31746));
#5941=EDGE_LOOP('',(#31747,#31748,#31749,#31750));
#5942=EDGE_LOOP('',(#31751,#31752,#31753,#31754));
#5943=EDGE_LOOP('',(#31755,#31756,#31757));
#5944=EDGE_LOOP('',(#31758,#31759,#31760,#31761));
#5945=EDGE_LOOP('',(#31762,#31763,#31764));
#5946=EDGE_LOOP('',(#31765,#31766,#31767));
#5947=EDGE_LOOP('',(#31768,#31769,#31770,#31771,#31772));
#5948=EDGE_LOOP('',(#31773,#31774,#31775,#31776));
#5949=EDGE_LOOP('',(#31777,#31778,#31779,#31780,#31781));
#5950=EDGE_LOOP('',(#31782,#31783,#31784));
#5951=EDGE_LOOP('',(#31785,#31786,#31787,#31788));
#5952=EDGE_LOOP('',(#31789,#31790,#31791,#31792,#31793,#31794));
#5953=EDGE_LOOP('',(#31795,#31796,#31797));
#5954=EDGE_LOOP('',(#31798,#31799,#31800,#31801,#31802));
#5955=EDGE_LOOP('',(#31803,#31804,#31805,#31806,#31807));
#5956=EDGE_LOOP('',(#31808,#31809,#31810,#31811,#31812));
#8247=CIRCLE('',#43000,17.8828427124746);
#8248=CIRCLE('',#43001,17.8828427124746);
#8249=CIRCLE('',#43002,0.4);
#8250=CIRCLE('',#43003,18.);
#8251=CIRCLE('',#43004,18.);
#8252=CIRCLE('',#43006,18.);
#8253=CIRCLE('',#43007,18.);
#8254=CIRCLE('',#43009,17.7171572875254);
#8255=CIRCLE('',#43010,17.7171572875254);
#8256=CIRCLE('',#43012,0.4);
#8257=CIRCLE('',#43013,17.6);
#8258=CIRCLE('',#43015,0.4);
#8259=CIRCLE('',#43016,0.4);
#8260=CIRCLE('',#43017,0.4);
#8261=CIRCLE('',#43018,0.4);
#8262=CIRCLE('',#43019,0.4);
#8263=CIRCLE('',#43020,0.4);
#8264=CIRCLE('',#43021,0.4);
#8265=CIRCLE('',#43022,0.4);
#8266=CIRCLE('',#43023,0.4);
#8267=CIRCLE('',#43024,0.4);
#8268=CIRCLE('',#43025,0.4);
#8269=CIRCLE('',#43026,0.4);
#8270=CIRCLE('',#43028,0.400000000000001);
#8271=CIRCLE('',#43029,0.4);
#8272=CIRCLE('',#43030,0.4);
#8273=CIRCLE('',#43035,17.4343145750508);
#8274=CIRCLE('',#43036,0.4);
#8275=CIRCLE('',#43038,11.45);
#8276=CIRCLE('',#43040,11.05);
#8277=CIRCLE('',#43041,11.05);
#8278=CIRCLE('',#43042,0.4);
#8279=CIRCLE('',#43044,11.05);
#8280=CIRCLE('',#43045,11.05);
#8281=CIRCLE('',#43047,11.182414107351);
#8282=CIRCLE('',#43048,11.182414107351);
#8283=CIRCLE('',#43049,0.4);
#8284=CIRCLE('',#43051,11.8247973983321);
#8285=CIRCLE('',#43052,11.8247973983321);
#8286=CIRCLE('',#43054,0.399999999999997);
#8287=CIRCLE('',#43055,0.4);
#8288=CIRCLE('',#43056,0.399999999999999);
#8289=CIRCLE('',#43058,0.4);
#8290=CIRCLE('',#43060,0.4);
#8291=CIRCLE('',#43062,0.4);
#8292=CIRCLE('',#43064,0.400000000000001);
#8293=CIRCLE('',#43066,15.8256568245417);
#8294=CIRCLE('',#43068,15.5589388807538);
#8295=CIRCLE('',#43069,0.4);
#8296=CIRCLE('',#43071,15.5589388807538);
#8297=CIRCLE('',#43072,15.5589388807538);
#8298=CIRCLE('',#43073,15.5589388807538);
#8299=CIRCLE('',#43074,15.5589388807538);
#8300=CIRCLE('',#43075,15.5589388807538);
#8301=CIRCLE('',#43076,15.5589388807538);
#8302=CIRCLE('',#43077,15.5589388807538);
#8303=CIRCLE('',#43078,15.5589388807538);
#8304=CIRCLE('',#43079,15.5589388807538);
#8305=CIRCLE('',#43080,15.5589388807538);
#8306=CIRCLE('',#43081,15.5589388807538);
#8307=CIRCLE('',#43082,12.0923832909811);
#8308=CIRCLE('',#43084,0.4);
#8309=CIRCLE('',#43085,0.4);
#8310=CIRCLE('',#43086,0.4);
#8311=CIRCLE('',#43087,0.4);
#8312=CIRCLE('',#43089,0.4);
#8313=CIRCLE('',#43091,0.399999999999088);
#8314=CIRCLE('',#43092,0.399999999999999);
#8315=CIRCLE('',#43094,0.4);
#8316=CIRCLE('',#43096,0.4);
#8317=CIRCLE('',#43101,0.4);
#8318=CIRCLE('',#43103,0.399999999999024);
#8319=CIRCLE('',#43104,0.4);
#8320=CIRCLE('',#43106,0.4);
#8321=CIRCLE('',#43108,0.399999999999998);
#8322=CIRCLE('',#43110,0.400000000000001);
#8323=CIRCLE('',#43112,15.8256568245417);
#8324=CIRCLE('',#43113,0.4);
#8325=CIRCLE('',#43115,0.399999999999999);
#8326=CIRCLE('',#43118,0.4);
#8327=CIRCLE('',#43120,0.4);
#8328=CIRCLE('',#43122,0.4);
#8329=CIRCLE('',#43125,15.8256568245417);
#8330=CIRCLE('',#43128,15.8256568245417);
#8331=CIRCLE('',#43136,0.399999999999997);
#8332=CIRCLE('',#43139,0.4);
#8333=CIRCLE('',#43140,0.399999999999091);
#8334=CIRCLE('',#43141,0.399999999999999);
#8335=CIRCLE('',#43143,0.4);
#8336=CIRCLE('',#43144,0.399999999999998);
#8337=CIRCLE('',#43146,0.4);
#8338=CIRCLE('',#43150,15.8256568245417);
#8339=CIRCLE('',#43151,0.4);
#8340=CIRCLE('',#43154,0.4);
#8341=CIRCLE('',#43156,0.399999999999997);
#8342=CIRCLE('',#43159,0.4);
#8343=CIRCLE('',#43161,0.4);
#8344=CIRCLE('',#43162,0.4);
#8345=CIRCLE('',#43163,0.4);
#8346=CIRCLE('',#43165,0.4);
#8347=CIRCLE('',#43166,0.399999999998833);
#8348=CIRCLE('',#43168,0.4);
#8349=CIRCLE('',#43171,0.4);
#8350=CIRCLE('',#43173,0.4);
#8351=CIRCLE('',#43174,0.399999999999999);
#8352=CIRCLE('',#43175,0.399999999999999);
#8353=CIRCLE('',#43177,0.399999999999999);
#8354=CIRCLE('',#43178,0.399999999998823);
#8355=CIRCLE('',#43180,0.4);
#8356=CIRCLE('',#43182,0.4);
#8357=CIRCLE('',#43184,0.4);
#8358=CIRCLE('',#43186,0.4);
#8359=CIRCLE('',#43188,0.4);
#8360=CIRCLE('',#43192,15.8256568245417);
#8361=CIRCLE('',#43195,15.8256568245417);
#8362=CIRCLE('',#43201,0.399999999999997);
#8363=CIRCLE('',#43204,0.4);
#8364=CIRCLE('',#43206,15.8256568245417);
#8365=CIRCLE('',#43211,0.400000000000002);
#8366=CIRCLE('',#43212,0.400000000000001);
#8367=CIRCLE('',#43213,0.400000000000001);
#8368=CIRCLE('',#43216,0.4);
#8369=CIRCLE('',#43217,0.4);
#8370=CIRCLE('',#43219,0.4);
#8371=CIRCLE('',#43222,0.4);
#8372=CIRCLE('',#43223,15.8256568245417);
#8373=CIRCLE('',#43224,0.399999999999999);
#8374=CIRCLE('',#43227,0.399999999999998);
#8375=CIRCLE('',#43232,0.4);
#8376=CIRCLE('',#43233,0.400000000000001);
#8377=CIRCLE('',#43234,0.400000000000001);
#8378=CIRCLE('',#43238,0.4);
#8379=CIRCLE('',#43239,0.399999999999999);
#8380=CIRCLE('',#43240,0.4);
#8381=CIRCLE('',#43245,0.4);
#8382=CIRCLE('',#43246,0.400000000000001);
#8383=CIRCLE('',#43247,0.399999999999998);
#8384=CIRCLE('',#43250,0.4);
#8385=CIRCLE('',#43251,0.400000000000002);
#8386=CIRCLE('',#43253,0.4);
#8387=CIRCLE('',#43255,0.4);
#8388=CIRCLE('',#43256,15.8256568245417);
#8389=CIRCLE('',#43257,0.4);
#8390=CIRCLE('',#43260,0.4);
#8391=CIRCLE('',#43265,15.8256568245417);
#8392=CIRCLE('',#43269,15.8256568245417);
#10073=B_SPLINE_CURVE_WITH_KNOTS('',3,(#77238,#77239,#77240,#77241),
 .UNSPECIFIED.,.F.,.F.,(4,4),(-0.597949259053295,-0.238859576382585),
 .UNSPECIFIED.);
#10074=B_SPLINE_CURVE_WITH_KNOTS('',3,(#77264,#77265,#77266,#77267),
 .UNSPECIFIED.,.F.,.F.,(4,4),(0.238859576382585,0.47008310880495),
 .UNSPECIFIED.);
#10075=B_SPLINE_CURVE_WITH_KNOTS('',3,(#77269,#77270,#77271,#77272,#77273,
#77274),.UNSPECIFIED.,.F.,.F.,(4,2,4),(-0.000645109744100447,0.,0.119683314027494),
 .UNSPECIFIED.);
#10076=B_SPLINE_CURVE_WITH_KNOTS('',3,(#77275,#77276,#77277,#77278,#77279,
#77280,#77281),.UNSPECIFIED.,.F.,.F.,(4,3,4),(0.0616297557035894,0.0751520318454544,
0.0767347622996508),.UNSPECIFIED.);
#10077=B_SPLINE_CURVE_WITH_KNOTS('',3,(#77299,#77300,#77301,#77302),
 .UNSPECIFIED.,.F.,.F.,(4,4),(-0.520475215840057,-0.161384884357676),
 .UNSPECIFIED.);
#10078=B_SPLINE_CURVE_WITH_KNOTS('',3,(#77304,#77305,#77306,#77307,#77308,
#77309,#77310),.UNSPECIFIED.,.F.,.F.,(4,3,4),(0.,0.0199523139593889,0.0221863619808638),
 .UNSPECIFIED.);
#10079=B_SPLINE_CURVE_WITH_KNOTS('',3,(#77312,#77313,#77314,#77315,#77316,
#77317),.UNSPECIFIED.,.F.,.F.,(4,2,4),(0.,0.0960567002189493,0.096575729291192),
 .UNSPECIFIED.);
#10080=B_SPLINE_CURVE_WITH_KNOTS('',3,(#77318,#77319,#77320,#77321),
 .UNSPECIFIED.,.F.,.F.,(4,4),(0.289251501550698,0.520475215840057),
 .UNSPECIFIED.);
#10081=B_SPLINE_CURVE_WITH_KNOTS('',3,(#77378,#77379,#77380,#77381),
 .UNSPECIFIED.,.F.,.F.,(4,4),(-0.231241687907805,0.),.UNSPECIFIED.);
#10082=B_SPLINE_CURVE_WITH_KNOTS('',3,(#77384,#77385,#77386,#77387),
 .UNSPECIFIED.,.F.,.F.,(4,4),(0.,0.231241687907805),.UNSPECIFIED.);
#10083=B_SPLINE_CURVE_WITH_KNOTS('',3,(#77399,#77400,#77401,#77402),
 .UNSPECIFIED.,.F.,.F.,(4,4),(-0.464164679032266,-0.232923065268537),
 .UNSPECIFIED.);
#10084=B_SPLINE_CURVE_WITH_KNOTS('',3,(#77423,#77424,#77425,#77426),
 .UNSPECIFIED.,.F.,.F.,(4,4),(0.232923065268537,0.464164679032266),
 .UNSPECIFIED.);
#10085=B_SPLINE_CURVE_WITH_KNOTS('',3,(#77453,#77454,#77455,#77456,#77457,
#77458,#77459),.UNSPECIFIED.,.F.,.F.,(4,3,4),(0.0616297557036194,0.0751520318454991,
0.0767347622996923),.UNSPECIFIED.);
#10086=B_SPLINE_CURVE_WITH_KNOTS('',3,(#77463,#77464,#77465,#77466,#77467,
#77468,#77469),.UNSPECIFIED.,.F.,.F.,(4,3,4),(0.,0.0199678703942285,0.0221878858471501),
 .UNSPECIFIED.);
#10087=B_SPLINE_CURVE_WITH_KNOTS('',3,(#77475,#77476,#77477,#77478,#77479,
#77480,#77481),.UNSPECIFIED.,.F.,.F.,(4,3,4),(0.0616297334270067,0.0751521942970439,
0.0767343333817494),.UNSPECIFIED.);
#10088=B_SPLINE_CURVE_WITH_KNOTS('',3,(#77485,#77486,#77487,#77488,#77489,
#77490,#77491),.UNSPECIFIED.,.F.,.F.,(4,3,4),(0.,0.0199653259285015,0.0221876721414005),
 .UNSPECIFIED.);
#10089=B_SPLINE_CURVE_WITH_KNOTS('',3,(#77558,#77559,#77560,#77561),
 .UNSPECIFIED.,.F.,.F.,(4,4),(-0.23124168790661,0.),.UNSPECIFIED.);
#10090=B_SPLINE_CURVE_WITH_KNOTS('',3,(#77562,#77563,#77564,#77565),
 .UNSPECIFIED.,.F.,.F.,(4,4),(0.,0.23124168790661),.UNSPECIFIED.);
#10091=B_SPLINE_CURVE_WITH_KNOTS('',3,(#77591,#77592,#77593,#77594),
 .UNSPECIFIED.,.F.,.F.,(4,4),(-0.2312416879078,0.),.UNSPECIFIED.);
#10092=B_SPLINE_CURVE_WITH_KNOTS('',3,(#77596,#77597,#77598,#77599),
 .UNSPECIFIED.,.F.,.F.,(4,4),(0.,0.2312416879078),.UNSPECIFIED.);
#10093=B_SPLINE_CURVE_WITH_KNOTS('',3,(#77636,#77637,#77638,#77639),
 .UNSPECIFIED.,.F.,.F.,(4,4),(-0.231241687907749,0.),.UNSPECIFIED.);
#10094=B_SPLINE_CURVE_WITH_KNOTS('',3,(#77642,#77643,#77644,#77645),
 .UNSPECIFIED.,.F.,.F.,(4,4),(0.,0.231241687907749),.UNSPECIFIED.);
#10095=B_SPLINE_CURVE_WITH_KNOTS('',3,(#77660,#77661,#77662,#77663),
 .UNSPECIFIED.,.F.,.F.,(4,4),(0.,0.231241350797188),.UNSPECIFIED.);
#10096=B_SPLINE_CURVE_WITH_KNOTS('',3,(#77681,#77682,#77683,#77684),
 .UNSPECIFIED.,.F.,.F.,(4,4),(-0.231241350797188,0.),.UNSPECIFIED.);
#10097=B_SPLINE_CURVE_WITH_KNOTS('',3,(#77696,#77697,#77698,#77699,#77700,
#77701,#77702,#77703,#77704,#77705,#77706,#77707,#77708,#77709,#77710,#77711,
#77712,#77713,#77714,#77715,#77716,#77717,#77718,#77719,#77720),
 .UNSPECIFIED.,.F.,.F.,(4,3,3,3,3,3,3,3,4),(-0.0439263344697962,-0.0437155216588433,
-0.035784713835945,-0.0298801140099492,-0.0225440807053907,-0.0163325858112043,
-0.00963041157950245,-0.00335144354243791,0.),.UNSPECIFIED.);
#10098=B_SPLINE_CURVE_WITH_KNOTS('',3,(#77721,#77722,#77723,#77724),
 .UNSPECIFIED.,.F.,.F.,(4,4),(0.0892538276575492,0.0934531910588508),
 .UNSPECIFIED.);
#10099=B_SPLINE_CURVE_WITH_KNOTS('',3,(#77742,#77743,#77744,#77745),
 .UNSPECIFIED.,.F.,.F.,(4,4),(-0.231242054178833,0.),.UNSPECIFIED.);
#10100=B_SPLINE_CURVE_WITH_KNOTS('',3,(#77748,#77749,#77750,#77751),
 .UNSPECIFIED.,.F.,.F.,(4,4),(0.,0.252215655062094),.UNSPECIFIED.);
#10101=B_SPLINE_CURVE_WITH_KNOTS('',3,(#77768,#77769,#77770,#77771,#77772,
#77773,#77774,#77775,#77776,#77777,#77778,#77779,#77780,#77781,#77782),
 .UNSPECIFIED.,.F.,.F.,(4,2,2,2,2,3,4),(0.479368947310773,0.479651170741328,
0.511663463377373,0.527669609695395,0.535672682854406,0.543675756013417,
0.545416548676313),.UNSPECIFIED.);
#10102=B_SPLINE_CURVE_WITH_KNOTS('',3,(#77784,#77785,#77786,#77787,#77788,
#77789,#77790,#77791),.UNSPECIFIED.,.F.,.F.,(4,2,2,4),(-0.0295125309642771,
-0.0147905162628861,0.,0.000289490369011506),.UNSPECIFIED.);
#10103=B_SPLINE_CURVE_WITH_KNOTS('',3,(#77826,#77827,#77828,#77829),
 .UNSPECIFIED.,.F.,.F.,(4,4),(-0.231241687907802,0.),.UNSPECIFIED.);
#10104=B_SPLINE_CURVE_WITH_KNOTS('',3,(#77832,#77833,#77834,#77835),
 .UNSPECIFIED.,.F.,.F.,(4,4),(0.,0.231241687907802),.UNSPECIFIED.);
#10105=B_SPLINE_CURVE_WITH_KNOTS('',3,(#77850,#77851,#77852,#77853),
 .UNSPECIFIED.,.F.,.F.,(4,4),(0.,0.231241586165377),.UNSPECIFIED.);
#10106=B_SPLINE_CURVE_WITH_KNOTS('',3,(#77874,#77875,#77876,#77877),
 .UNSPECIFIED.,.F.,.F.,(4,4),(-0.231241586165377,0.),.UNSPECIFIED.);
#10107=B_SPLINE_CURVE_WITH_KNOTS('',3,(#77915,#77916,#77917,#77918),
 .UNSPECIFIED.,.F.,.F.,(4,4),(-0.23124114363781,0.),.UNSPECIFIED.);
#10108=B_SPLINE_CURVE_WITH_KNOTS('',3,(#77921,#77922,#77923,#77924),
 .UNSPECIFIED.,.F.,.F.,(4,4),(0.,0.23124114363781),.UNSPECIFIED.);
#10109=B_SPLINE_CURVE_WITH_KNOTS('',3,(#77942,#77943,#77944,#77945),
 .UNSPECIFIED.,.F.,.F.,(4,4),(0.228586915697378,0.459828059335187),
 .UNSPECIFIED.);
#10110=B_SPLINE_CURVE_WITH_KNOTS('',3,(#77947,#77948,#77949,#77950),
 .UNSPECIFIED.,.F.,.F.,(4,4),(-0.459828059335187,-0.228586915820151),
 .UNSPECIFIED.);
#10111=B_SPLINE_CURVE_WITH_KNOTS('',3,(#77987,#77988,#77989,#77990),
 .UNSPECIFIED.,.F.,.F.,(4,4),(-0.231241350797186,0.),.UNSPECIFIED.);
#10112=B_SPLINE_CURVE_WITH_KNOTS('',3,(#77993,#77994,#77995,#77996),
 .UNSPECIFIED.,.F.,.F.,(4,4),(0.,0.231241350797186),.UNSPECIFIED.);
#10113=B_SPLINE_CURVE_WITH_KNOTS('',3,(#78014,#78015,#78016,#78017),
 .UNSPECIFIED.,.F.,.F.,(4,4),(0.215800706400213,0.447042292565588),
 .UNSPECIFIED.);
#10114=B_SPLINE_CURVE_WITH_KNOTS('',3,(#78019,#78020,#78021,#78022),
 .UNSPECIFIED.,.F.,.F.,(4,4),(-0.447042292565588,-0.215800706400213),
 .UNSPECIFIED.);
#10115=B_SPLINE_CURVE_WITH_KNOTS('',3,(#78071,#78072,#78073,#78074),
 .UNSPECIFIED.,.F.,.F.,(4,4),(-0.459827831361922,-0.228585906851782),
 .UNSPECIFIED.);
#10116=B_SPLINE_CURVE_WITH_KNOTS('',3,(#78093,#78094,#78095,#78096),
 .UNSPECIFIED.,.F.,.F.,(4,4),(0.228585906851782,0.459827831361922),
 .UNSPECIFIED.);
#10117=B_SPLINE_CURVE_WITH_KNOTS('',3,(#78115,#78116,#78117,#78118),
 .UNSPECIFIED.,.F.,.F.,(4,4),(-0.520475100360999,-0.289233280455309),
 .UNSPECIFIED.);
#10118=B_SPLINE_CURVE_WITH_KNOTS('',3,(#78121,#78122,#78123,#78124),
 .UNSPECIFIED.,.F.,.F.,(4,4),(0.289233280455309,0.520475100360999),
 .UNSPECIFIED.);
#10119=B_SPLINE_CURVE_WITH_KNOTS('',3,(#78152,#78153,#78154,#78155),
 .UNSPECIFIED.,.F.,.F.,(4,4),(-0.587676103485633,-0.228585906851781),
 .UNSPECIFIED.);
#10120=B_SPLINE_CURVE_WITH_KNOTS('',3,(#78174,#78175,#78176,#78177),
 .UNSPECIFIED.,.F.,.F.,(4,4),(0.228585906851781,0.459809595893694),
 .UNSPECIFIED.);
#10121=B_SPLINE_CURVE_WITH_KNOTS('',3,(#78178,#78179,#78180,#78181,#78182,
#78183),.UNSPECIFIED.,.F.,.F.,(4,2,4),(-0.000645327069758885,0.,0.119683098516029),
 .UNSPECIFIED.);
#10122=B_SPLINE_CURVE_WITH_KNOTS('',3,(#78200,#78201,#78202,#78203),
 .UNSPECIFIED.,.F.,.F.,(4,4),(-0.516463029416307,-0.157372832782455),
 .UNSPECIFIED.);
#10123=B_SPLINE_CURVE_WITH_KNOTS('',3,(#78205,#78206,#78207,#78208,#78209,
#78210),.UNSPECIFIED.,.F.,.F.,(4,2,4),(0.,0.0960578455735924,0.0965757861080569),
 .UNSPECIFIED.);
#10124=B_SPLINE_CURVE_WITH_KNOTS('',3,(#78211,#78212,#78213,#78214),
 .UNSPECIFIED.,.F.,.F.,(4,4),(0.285239340374395,0.516463029416307),
 .UNSPECIFIED.);
#10125=B_SPLINE_CURVE_WITH_KNOTS('',3,(#78226,#78227,#78228,#78229),
 .UNSPECIFIED.,.F.,.F.,(4,4),(-0.597949259053296,-0.238859576382585),
 .UNSPECIFIED.);
#10126=B_SPLINE_CURVE_WITH_KNOTS('',3,(#78250,#78251,#78252,#78253),
 .UNSPECIFIED.,.F.,.F.,(4,4),(0.238859576382585,0.470083108804951),
 .UNSPECIFIED.);
#10127=B_SPLINE_CURVE_WITH_KNOTS('',3,(#78254,#78255,#78256,#78257,#78258,
#78259),.UNSPECIFIED.,.F.,.F.,(4,2,4),(-0.000645109738815446,0.,0.119683312515737),
 .UNSPECIFIED.);
#10128=B_SPLINE_CURVE_WITH_KNOTS('',3,(#78276,#78277,#78278,#78279),
 .UNSPECIFIED.,.F.,.F.,(4,4),(-0.503986701734181,-0.14489400298759),
 .UNSPECIFIED.);
#10129=B_SPLINE_CURVE_WITH_KNOTS('',3,(#78281,#78282,#78283,#78284,#78285,
#78286),.UNSPECIFIED.,.F.,.F.,(4,2,4),(0.,0.0960580344299204,0.0965757964360946),
 .UNSPECIFIED.);
#10130=B_SPLINE_CURVE_WITH_KNOTS('',3,(#78287,#78288,#78289,#78290),
 .UNSPECIFIED.,.F.,.F.,(4,4),(0.272760383782263,0.503986701734181),
 .UNSPECIFIED.);
#10131=B_SPLINE_CURVE_WITH_KNOTS('',3,(#78303,#78304,#78305,#78306),
 .UNSPECIFIED.,.F.,.F.,(4,4),(-0.464164679032267,-0.232923065268538),
 .UNSPECIFIED.);
#10132=B_SPLINE_CURVE_WITH_KNOTS('',3,(#78325,#78326,#78327,#78328),
 .UNSPECIFIED.,.F.,.F.,(4,4),(0.232923065268538,0.464164679032267),
 .UNSPECIFIED.);
#10133=B_SPLINE_CURVE_WITH_KNOTS('',3,(#78347,#78348,#78349,#78350),
 .UNSPECIFIED.,.F.,.F.,(4,4),(-0.502582702411899,-0.27134084970268),
 .UNSPECIFIED.);
#10134=B_SPLINE_CURVE_WITH_KNOTS('',3,(#78353,#78354,#78355,#78356),
 .UNSPECIFIED.,.F.,.F.,(4,4),(0.27134084970268,0.502582702411899),
 .UNSPECIFIED.);
#11393=LINE('',#77139,#13887);
#11394=LINE('',#77147,#13888);
#11395=LINE('',#77156,#13889);
#11396=LINE('',#77158,#13890);
#11397=LINE('',#77162,#13891);
#11398=LINE('',#77164,#13892);
#11399=LINE('',#77168,#13893);
#11400=LINE('',#77170,#13894);
#11401=LINE('',#77174,#13895);
#11402=LINE('',#77176,#13896);
#11403=LINE('',#77180,#13897);
#11404=LINE('',#77182,#13898);
#11405=LINE('',#77186,#13899);
#11406=LINE('',#77188,#13900);
#11407=LINE('',#77192,#13901);
#11408=LINE('',#77194,#13902);
#11409=LINE('',#77198,#13903);
#11410=LINE('',#77200,#13904);
#11411=LINE('',#77204,#13905);
#11412=LINE('',#77206,#13906);
#11413=LINE('',#77210,#13907);
#11414=LINE('',#77212,#13908);
#11415=LINE('',#77216,#13909);
#11416=LINE('',#77218,#13910);
#11417=LINE('',#77222,#13911);
#11418=LINE('',#77224,#13912);
#11419=LINE('',#77234,#13913);
#11420=LINE('',#77235,#13914);
#11421=LINE('',#77243,#13915);
#11422=LINE('',#77246,#13916);
#11423=LINE('',#77337,#13917);
#11424=LINE('',#77351,#13918);
#11425=LINE('',#77357,#13919);
#11426=LINE('',#77358,#13920);
#11427=LINE('',#77391,#13921);
#11428=LINE('',#77392,#13922);
#11429=LINE('',#77404,#13923);
#11430=LINE('',#77405,#13924);
#11431=LINE('',#77437,#13925);
#11432=LINE('',#77439,#13926);
#11433=LINE('',#77443,#13927);
#11434=LINE('',#77445,#13928);
#11435=LINE('',#77449,#13929);
#11436=LINE('',#77451,#13930);
#11437=LINE('',#77471,#13931);
#11438=LINE('',#77473,#13932);
#11439=LINE('',#77493,#13933);
#11440=LINE('',#77495,#13934);
#11441=LINE('',#77499,#13935);
#11442=LINE('',#77501,#13936);
#11443=LINE('',#77505,#13937);
#11444=LINE('',#77507,#13938);
#11445=LINE('',#77511,#13939);
#11446=LINE('',#77513,#13940);
#11447=LINE('',#77517,#13941);
#11448=LINE('',#77519,#13942);
#11449=LINE('',#77523,#13943);
#11450=LINE('',#77525,#13944);
#11451=LINE('',#77529,#13945);
#11452=LINE('',#77530,#13946);
#11453=LINE('',#77571,#13947);
#11454=LINE('',#77605,#13948);
#11455=LINE('',#77606,#13949);
#11456=LINE('',#77608,#13950);
#11457=LINE('',#77610,#13951);
#11458=LINE('',#77616,#13952);
#11459=LINE('',#77651,#13953);
#11460=LINE('',#77652,#13954);
#11461=LINE('',#77688,#13955);
#11462=LINE('',#77689,#13956);
#11463=LINE('',#77692,#13957);
#11464=LINE('',#77694,#13958);
#11465=LINE('',#77754,#13959);
#11466=LINE('',#77763,#13960);
#11467=LINE('',#77764,#13961);
#11468=LINE('',#77802,#13962);
#11469=LINE('',#77844,#13963);
#11470=LINE('',#77855,#13964);
#11471=LINE('',#77856,#13965);
#11472=LINE('',#77882,#13966);
#11473=LINE('',#77887,#13967);
#11474=LINE('',#77896,#13968);
#11475=LINE('',#77897,#13969);
#11476=LINE('',#77954,#13970);
#11477=LINE('',#77959,#13971);
#11478=LINE('',#77968,#13972);
#11479=LINE('',#77969,#13973);
#11480=LINE('',#78025,#13974);
#11481=LINE('',#78044,#13975);
#11482=LINE('',#78046,#13976);
#11483=LINE('',#78056,#13977);
#11484=LINE('',#78067,#13978);
#11485=LINE('',#78068,#13979);
#11486=LINE('',#78075,#13980);
#11487=LINE('',#78128,#13981);
#11488=LINE('',#78140,#13982);
#11489=LINE('',#78149,#13983);
#11490=LINE('',#78150,#13984);
#11491=LINE('',#78156,#13985);
#11492=LINE('',#78223,#13986);
#11493=LINE('',#78224,#13987);
#11494=LINE('',#78232,#13988);
#11495=LINE('',#78299,#13989);
#11496=LINE('',#78300,#13990);
#11497=LINE('',#78307,#13991);
#11498=LINE('',#78359,#13992);
#13887=VECTOR('',#51243,18.);
#13888=VECTOR('',#51252,17.8);
#13889=VECTOR('',#51263,10.);
#13890=VECTOR('',#51264,10.);
#13891=VECTOR('',#51267,10.);
#13892=VECTOR('',#51268,10.);
#13893=VECTOR('',#51271,10.);
#13894=VECTOR('',#51272,10.);
#13895=VECTOR('',#51275,10.);
#13896=VECTOR('',#51276,10.);
#13897=VECTOR('',#51279,10.);
#13898=VECTOR('',#51280,10.);
#13899=VECTOR('',#51283,10.);
#13900=VECTOR('',#51284,10.);
#13901=VECTOR('',#51287,10.);
#13902=VECTOR('',#51288,10.);
#13903=VECTOR('',#51291,10.);
#13904=VECTOR('',#51292,10.);
#13905=VECTOR('',#51295,10.);
#13906=VECTOR('',#51296,10.);
#13907=VECTOR('',#51299,10.);
#13908=VECTOR('',#51300,10.);
#13909=VECTOR('',#51303,10.);
#13910=VECTOR('',#51304,10.);
#13911=VECTOR('',#51307,10.);
#13912=VECTOR('',#51308,10.);
#13913=VECTOR('',#51321,10.);
#13914=VECTOR('',#51322,10.);
#13915=VECTOR('',#51325,10.);
#13916=VECTOR('',#51328,10.);
#13917=VECTOR('',#51349,11.05);
#13918=VECTOR('',#51366,11.55);
#13919=VECTOR('',#51373,10.);
#13920=VECTOR('',#51374,10.);
#13921=VECTOR('',#51383,10.);
#13922=VECTOR('',#51384,10.);
#13923=VECTOR('',#51395,10.);
#13924=VECTOR('',#51396,10.);
#13925=VECTOR('',#51413,10.);
#13926=VECTOR('',#51414,10.);
#13927=VECTOR('',#51417,10.);
#13928=VECTOR('',#51418,10.);
#13929=VECTOR('',#51421,10.);
#13930=VECTOR('',#51422,10.);
#13931=VECTOR('',#51425,10.);
#13932=VECTOR('',#51426,10.);
#13933=VECTOR('',#51429,10.);
#13934=VECTOR('',#51430,10.);
#13935=VECTOR('',#51433,10.);
#13936=VECTOR('',#51434,10.);
#13937=VECTOR('',#51437,10.);
#13938=VECTOR('',#51438,10.);
#13939=VECTOR('',#51441,10.);
#13940=VECTOR('',#51442,10.);
#13941=VECTOR('',#51445,10.);
#13942=VECTOR('',#51446,10.);
#13943=VECTOR('',#51449,10.);
#13944=VECTOR('',#51450,10.);
#13945=VECTOR('',#51453,10.);
#13946=VECTOR('',#51454,10.);
#13947=VECTOR('',#51473,10.);
#13948=VECTOR('',#51488,10.);
#13949=VECTOR('',#51489,10.);
#13950=VECTOR('',#51492,10.);
#13951=VECTOR('',#51495,10.);
#13952=VECTOR('',#51502,10.);
#13953=VECTOR('',#51515,10.);
#13954=VECTOR('',#51516,10.);
#13955=VECTOR('',#51533,10.);
#13956=VECTOR('',#51534,10.);
#13957=VECTOR('',#51537,10.);
#13958=VECTOR('',#51538,10.);
#13959=VECTOR('',#51545,10.);
#13960=VECTOR('',#51552,10.);
#13961=VECTOR('',#51553,10.);
#13962=VECTOR('',#51578,10.);
#13963=VECTOR('',#51605,10.);
#13964=VECTOR('',#51616,10.);
#13965=VECTOR('',#51617,10.);
#13966=VECTOR('',#51622,10.);
#13967=VECTOR('',#51631,10.);
#13968=VECTOR('',#51642,10.);
#13969=VECTOR('',#51643,10.);
#13970=VECTOR('',#51650,10.);
#13971=VECTOR('',#51659,10.);
#13972=VECTOR('',#51670,10.);
#13973=VECTOR('',#51671,10.);
#13974=VECTOR('',#51680,10.);
#13975=VECTOR('',#51717,10.);
#13976=VECTOR('',#51720,10.);
#13977=VECTOR('',#51737,10.);
#13978=VECTOR('',#51752,10.);
#13979=VECTOR('',#51753,10.);
#13980=VECTOR('',#51756,10.);
#13981=VECTOR('',#51765,10.);
#13982=VECTOR('',#51788,10.);
#13983=VECTOR('',#51799,10.);
#13984=VECTOR('',#51800,10.);
#13985=VECTOR('',#51803,10.);
#13986=VECTOR('',#51814,10.);
#13987=VECTOR('',#51815,10.);
#13988=VECTOR('',#51820,10.);
#13989=VECTOR('',#51831,10.);
#13990=VECTOR('',#51832,10.);
#13991=VECTOR('',#51835,10.);
#13992=VECTOR('',#51844,10.);
#17114=VERTEX_POINT('',#77128);
#17115=VERTEX_POINT('',#77129);
#17116=VERTEX_POINT('',#77132);
#17117=VERTEX_POINT('',#77134);
#17118=VERTEX_POINT('',#77138);
#17119=VERTEX_POINT('',#77140);
#17120=VERTEX_POINT('',#77144);
#17121=VERTEX_POINT('',#77145);
#17122=VERTEX_POINT('',#77150);
#17123=VERTEX_POINT('',#77154);
#17124=VERTEX_POINT('',#77155);
#17125=VERTEX_POINT('',#77157);
#17126=VERTEX_POINT('',#77159);
#17127=VERTEX_POINT('',#77161);
#17128=VERTEX_POINT('',#77163);
#17129=VERTEX_POINT('',#77165);
#17130=VERTEX_POINT('',#77167);
#17131=VERTEX_POINT('',#77169);
#17132=VERTEX_POINT('',#77171);
#17133=VERTEX_POINT('',#77173);
#17134=VERTEX_POINT('',#77175);
#17135=VERTEX_POINT('',#77177);
#17136=VERTEX_POINT('',#77179);
#17137=VERTEX_POINT('',#77181);
#17138=VERTEX_POINT('',#77183);
#17139=VERTEX_POINT('',#77185);
#17140=VERTEX_POINT('',#77187);
#17141=VERTEX_POINT('',#77189);
#17142=VERTEX_POINT('',#77191);
#17143=VERTEX_POINT('',#77193);
#17144=VERTEX_POINT('',#77195);
#17145=VERTEX_POINT('',#77197);
#17146=VERTEX_POINT('',#77199);
#17147=VERTEX_POINT('',#77201);
#17148=VERTEX_POINT('',#77203);
#17149=VERTEX_POINT('',#77205);
#17150=VERTEX_POINT('',#77207);
#17151=VERTEX_POINT('',#77209);
#17152=VERTEX_POINT('',#77211);
#17153=VERTEX_POINT('',#77213);
#17154=VERTEX_POINT('',#77215);
#17155=VERTEX_POINT('',#77217);
#17156=VERTEX_POINT('',#77219);
#17157=VERTEX_POINT('',#77221);
#17158=VERTEX_POINT('',#77223);
#17159=VERTEX_POINT('',#77227);
#17160=VERTEX_POINT('',#77228);
#17161=VERTEX_POINT('',#77230);
#17162=VERTEX_POINT('',#77237);
#17163=VERTEX_POINT('',#77242);
#17164=VERTEX_POINT('',#77244);
#17165=VERTEX_POINT('',#77263);
#17166=VERTEX_POINT('',#77268);
#17167=VERTEX_POINT('',#77298);
#17168=VERTEX_POINT('',#77303);
#17169=VERTEX_POINT('',#77311);
#17170=VERTEX_POINT('',#77323);
#17171=VERTEX_POINT('',#77327);
#17172=VERTEX_POINT('',#77330);
#17173=VERTEX_POINT('',#77331);
#17174=VERTEX_POINT('',#77336);
#17175=VERTEX_POINT('',#77338);
#17176=VERTEX_POINT('',#77342);
#17177=VERTEX_POINT('',#77343);
#17178=VERTEX_POINT('',#77348);
#17179=VERTEX_POINT('',#77349);
#17180=VERTEX_POINT('',#77354);
#17181=VERTEX_POINT('',#77355);
#17182=VERTEX_POINT('',#77375);
#17183=VERTEX_POINT('',#77377);
#17184=VERTEX_POINT('',#77382);
#17185=VERTEX_POINT('',#77389);
#17186=VERTEX_POINT('',#77398);
#17187=VERTEX_POINT('',#77403);
#17188=VERTEX_POINT('',#77422);
#17189=VERTEX_POINT('',#77431);
#17190=VERTEX_POINT('',#77436);
#17191=VERTEX_POINT('',#77438);
#17192=VERTEX_POINT('',#77440);
#17193=VERTEX_POINT('',#77442);
#17194=VERTEX_POINT('',#77444);
#17195=VERTEX_POINT('',#77446);
#17196=VERTEX_POINT('',#77448);
#17197=VERTEX_POINT('',#77450);
#17198=VERTEX_POINT('',#77452);
#17199=VERTEX_POINT('',#77460);
#17200=VERTEX_POINT('',#77462);
#17201=VERTEX_POINT('',#77470);
#17202=VERTEX_POINT('',#77472);
#17203=VERTEX_POINT('',#77474);
#17204=VERTEX_POINT('',#77482);
#17205=VERTEX_POINT('',#77484);
#17206=VERTEX_POINT('',#77492);
#17207=VERTEX_POINT('',#77494);
#17208=VERTEX_POINT('',#77496);
#17209=VERTEX_POINT('',#77498);
#17210=VERTEX_POINT('',#77500);
#17211=VERTEX_POINT('',#77502);
#17212=VERTEX_POINT('',#77504);
#17213=VERTEX_POINT('',#77506);
#17214=VERTEX_POINT('',#77508);
#17215=VERTEX_POINT('',#77510);
#17216=VERTEX_POINT('',#77512);
#17217=VERTEX_POINT('',#77514);
#17218=VERTEX_POINT('',#77516);
#17219=VERTEX_POINT('',#77518);
#17220=VERTEX_POINT('',#77520);
#17221=VERTEX_POINT('',#77522);
#17222=VERTEX_POINT('',#77524);
#17223=VERTEX_POINT('',#77526);
#17224=VERTEX_POINT('',#77528);
#17225=VERTEX_POINT('',#77531);
#17226=VERTEX_POINT('',#77534);
#17227=VERTEX_POINT('',#77535);
#17228=VERTEX_POINT('',#77555);
#17229=VERTEX_POINT('',#77556);
#17230=VERTEX_POINT('',#77567);
#17231=VERTEX_POINT('',#77569);
#17232=VERTEX_POINT('',#77588);
#17233=VERTEX_POINT('',#77590);
#17234=VERTEX_POINT('',#77612);
#17235=VERTEX_POINT('',#77614);
#17236=VERTEX_POINT('',#77633);
#17237=VERTEX_POINT('',#77635);
#17238=VERTEX_POINT('',#77640);
#17239=VERTEX_POINT('',#77649);
#17240=VERTEX_POINT('',#77656);
#17241=VERTEX_POINT('',#77680);
#17242=VERTEX_POINT('',#77687);
#17243=VERTEX_POINT('',#77691);
#17244=VERTEX_POINT('',#77693);
#17245=VERTEX_POINT('',#77695);
#17246=VERTEX_POINT('',#77741);
#17247=VERTEX_POINT('',#77746);
#17248=VERTEX_POINT('',#77758);
#17249=VERTEX_POINT('',#77762);
#17250=VERTEX_POINT('',#77766);
#17251=VERTEX_POINT('',#77801);
#17252=VERTEX_POINT('',#77823);
#17253=VERTEX_POINT('',#77825);
#17254=VERTEX_POINT('',#77830);
#17255=VERTEX_POINT('',#77837);
#17256=VERTEX_POINT('',#77846);
#17257=VERTEX_POINT('',#77873);
#17258=VERTEX_POINT('',#77880);
#17259=VERTEX_POINT('',#77881);
#17260=VERTEX_POINT('',#77889);
#17261=VERTEX_POINT('',#77890);
#17262=VERTEX_POINT('',#77892);
#17263=VERTEX_POINT('',#77914);
#17264=VERTEX_POINT('',#77919);
#17265=VERTEX_POINT('',#77941);
#17266=VERTEX_POINT('',#77952);
#17267=VERTEX_POINT('',#77953);
#17268=VERTEX_POINT('',#77961);
#17269=VERTEX_POINT('',#77962);
#17270=VERTEX_POINT('',#77964);
#17271=VERTEX_POINT('',#77986);
#17272=VERTEX_POINT('',#77991);
#17273=VERTEX_POINT('',#78013);
#17274=VERTEX_POINT('',#78055);
#17275=VERTEX_POINT('',#78060);
#17276=VERTEX_POINT('',#78061);
#17277=VERTEX_POINT('',#78063);
#17278=VERTEX_POINT('',#78070);
#17279=VERTEX_POINT('',#78092);
#17280=VERTEX_POINT('',#78114);
#17281=VERTEX_POINT('',#78119);
#17282=VERTEX_POINT('',#78127);
#17283=VERTEX_POINT('',#78142);
#17284=VERTEX_POINT('',#78143);
#17285=VERTEX_POINT('',#78145);
#17286=VERTEX_POINT('',#78173);
#17287=VERTEX_POINT('',#78204);
#17288=VERTEX_POINT('',#78216);
#17289=VERTEX_POINT('',#78217);
#17290=VERTEX_POINT('',#78219);
#17291=VERTEX_POINT('',#78230);
#17292=VERTEX_POINT('',#78249);
#17293=VERTEX_POINT('',#78280);
#17294=VERTEX_POINT('',#78292);
#17295=VERTEX_POINT('',#78293);
#17296=VERTEX_POINT('',#78295);
#17297=VERTEX_POINT('',#78302);
#17298=VERTEX_POINT('',#78324);
#17299=VERTEX_POINT('',#78346);
#17300=VERTEX_POINT('',#78351);
#22092=EDGE_CURVE('',#17114,#17115,#8247,.T.);
#22093=EDGE_CURVE('',#17115,#17114,#8248,.T.);
#22094=EDGE_CURVE('',#17114,#17116,#8249,.T.);
#22095=EDGE_CURVE('',#17116,#17117,#8250,.T.);
#22096=EDGE_CURVE('',#17117,#17116,#8251,.T.);
#22097=EDGE_CURVE('',#17117,#17118,#11393,.T.);
#22098=EDGE_CURVE('',#17119,#17118,#8252,.T.);
#22099=EDGE_CURVE('',#17118,#17119,#8253,.T.);
#22100=EDGE_CURVE('',#17120,#17121,#8254,.T.);
#22101=EDGE_CURVE('',#17120,#17115,#11394,.T.);
#22102=EDGE_CURVE('',#17121,#17120,#8255,.T.);
#22103=EDGE_CURVE('',#17119,#17122,#8256,.T.);
#22104=EDGE_CURVE('',#17122,#17122,#8257,.T.);
#22105=EDGE_CURVE('',#17123,#17124,#11395,.T.);
#22106=EDGE_CURVE('',#17124,#17125,#11396,.T.);
#22107=EDGE_CURVE('',#17126,#17125,#8258,.F.);
#22108=EDGE_CURVE('',#17126,#17127,#11397,.T.);
#22109=EDGE_CURVE('',#17127,#17128,#11398,.T.);
#22110=EDGE_CURVE('',#17129,#17128,#8259,.F.);
#22111=EDGE_CURVE('',#17129,#17130,#11399,.T.);
#22112=EDGE_CURVE('',#17130,#17131,#11400,.T.);
#22113=EDGE_CURVE('',#17132,#17131,#8260,.F.);
#22114=EDGE_CURVE('',#17132,#17133,#11401,.T.);
#22115=EDGE_CURVE('',#17133,#17134,#11402,.T.);
#22116=EDGE_CURVE('',#17135,#17134,#8261,.F.);
#22117=EDGE_CURVE('',#17135,#17136,#11403,.T.);
#22118=EDGE_CURVE('',#17136,#17137,#11404,.T.);
#22119=EDGE_CURVE('',#17138,#17137,#8262,.F.);
#22120=EDGE_CURVE('',#17138,#17139,#11405,.T.);
#22121=EDGE_CURVE('',#17139,#17140,#11406,.T.);
#22122=EDGE_CURVE('',#17141,#17140,#8263,.F.);
#22123=EDGE_CURVE('',#17141,#17142,#11407,.T.);
#22124=EDGE_CURVE('',#17142,#17143,#11408,.T.);
#22125=EDGE_CURVE('',#17144,#17143,#8264,.F.);
#22126=EDGE_CURVE('',#17144,#17145,#11409,.T.);
#22127=EDGE_CURVE('',#17145,#17146,#11410,.T.);
#22128=EDGE_CURVE('',#17147,#17146,#8265,.F.);
#22129=EDGE_CURVE('',#17147,#17148,#11411,.T.);
#22130=EDGE_CURVE('',#17148,#17149,#11412,.T.);
#22131=EDGE_CURVE('',#17150,#17149,#8266,.F.);
#22132=EDGE_CURVE('',#17150,#17151,#11413,.T.);
#22133=EDGE_CURVE('',#17151,#17152,#11414,.T.);
#22134=EDGE_CURVE('',#17153,#17152,#8267,.F.);
#22135=EDGE_CURVE('',#17153,#17154,#11415,.T.);
#22136=EDGE_CURVE('',#17154,#17155,#11416,.T.);
#22137=EDGE_CURVE('',#17156,#17155,#8268,.F.);
#22138=EDGE_CURVE('',#17156,#17157,#11417,.T.);
#22139=EDGE_CURVE('',#17157,#17158,#11418,.T.);
#22140=EDGE_CURVE('',#17123,#17158,#8269,.F.);
#22141=EDGE_CURVE('',#17159,#17160,#8270,.T.);
#22142=EDGE_CURVE('',#17160,#17161,#8271,.T.);
#22143=EDGE_CURVE('',#17161,#17159,#8272,.T.);
#22144=EDGE_CURVE('',#17159,#17138,#11419,.T.);
#22145=EDGE_CURVE('',#17137,#17160,#11420,.T.);
#22146=EDGE_CURVE('',#17162,#17159,#10073,.T.);
#22147=EDGE_CURVE('',#17162,#17163,#11421,.T.);
#22148=EDGE_CURVE('',#17164,#17163,#211,.F.);
#22149=EDGE_CURVE('',#17164,#17139,#11422,.T.);
#22150=EDGE_CURVE('',#17161,#17165,#10074,.T.);
#22151=EDGE_CURVE('',#17165,#17166,#10075,.T.);
#22152=EDGE_CURVE('',#17166,#17162,#10076,.T.);
#22153=EDGE_CURVE('',#17160,#17167,#10077,.T.);
#22154=EDGE_CURVE('',#17167,#17168,#10078,.T.);
#22155=EDGE_CURVE('',#17168,#17169,#10079,.T.);
#22156=EDGE_CURVE('',#17169,#17161,#10080,.T.);
#22157=EDGE_CURVE('',#17170,#17170,#8273,.T.);
#22158=EDGE_CURVE('',#17170,#17121,#8274,.T.);
#22159=EDGE_CURVE('',#17171,#17171,#8275,.T.);
#22160=EDGE_CURVE('',#17172,#17173,#8276,.T.);
#22161=EDGE_CURVE('',#17173,#17172,#8277,.T.);
#22162=EDGE_CURVE('',#17172,#17171,#8278,.T.);
#22163=EDGE_CURVE('',#17173,#17174,#11423,.T.);
#22164=EDGE_CURVE('',#17175,#17174,#8279,.T.);
#22165=EDGE_CURVE('',#17174,#17175,#8280,.T.);
#22166=EDGE_CURVE('',#17176,#17177,#8281,.T.);
#22167=EDGE_CURVE('',#17177,#17176,#8282,.T.);
#22168=EDGE_CURVE('',#17176,#17175,#8283,.T.);
#22169=EDGE_CURVE('',#17178,#17179,#8284,.T.);
#22170=EDGE_CURVE('',#17178,#17177,#11424,.T.);
#22171=EDGE_CURVE('',#17179,#17178,#8285,.T.);
#22172=EDGE_CURVE('',#17180,#17181,#8286,.T.);
#22173=EDGE_CURVE('',#17181,#17141,#11425,.T.);
#22174=EDGE_CURVE('',#17140,#17180,#11426,.T.);
#22175=EDGE_CURVE('',#17182,#17180,#8287,.T.);
#22176=EDGE_CURVE('',#17180,#17183,#10081,.T.);
#22177=EDGE_CURVE('',#17183,#17184,#8288,.T.);
#22178=EDGE_CURVE('',#17184,#17182,#10082,.T.);
#22179=EDGE_CURVE('',#17185,#17183,#8289,.T.);
#22180=EDGE_CURVE('',#17183,#17164,#11427,.T.);
#22181=EDGE_CURVE('',#17163,#17185,#11428,.T.);
#22182=EDGE_CURVE('',#17185,#17184,#8290,.T.);
#22183=EDGE_CURVE('',#17182,#17181,#8291,.T.);
#22184=EDGE_CURVE('',#17186,#17181,#10083,.T.);
#22185=EDGE_CURVE('',#17187,#17186,#11429,.T.);
#22186=EDGE_CURVE('',#17187,#17142,#11430,.T.);
#22187=EDGE_CURVE('',#17182,#17188,#10084,.T.);
#22188=EDGE_CURVE('',#17186,#17188,#8292,.T.);
#22189=EDGE_CURVE('',#17188,#17184,#8293,.T.);
#22190=EDGE_CURVE('',#17185,#17189,#8294,.T.);
#22191=EDGE_CURVE('',#17189,#17188,#8295,.T.);
#22192=EDGE_CURVE('',#17168,#17166,#8296,.T.);
#22193=EDGE_CURVE('',#17190,#17167,#11431,.T.);
#22194=EDGE_CURVE('',#17191,#17190,#11432,.T.);
#22195=EDGE_CURVE('',#17192,#17191,#8297,.T.);
#22196=EDGE_CURVE('',#17193,#17192,#11433,.T.);
#22197=EDGE_CURVE('',#17194,#17193,#11434,.T.);
#22198=EDGE_CURVE('',#17195,#17194,#8298,.T.);
#22199=EDGE_CURVE('',#17196,#17195,#11435,.T.);
#22200=EDGE_CURVE('',#17197,#17196,#11436,.T.);
#22201=EDGE_CURVE('',#17198,#17197,#10085,.T.);
#22202=EDGE_CURVE('',#17199,#17198,#8299,.T.);
#22203=EDGE_CURVE('',#17200,#17199,#10086,.T.);
#22204=EDGE_CURVE('',#17201,#17200,#11437,.T.);
#22205=EDGE_CURVE('',#17202,#17201,#11438,.T.);
#22206=EDGE_CURVE('',#17203,#17202,#10087,.T.);
#22207=EDGE_CURVE('',#17204,#17203,#8300,.T.);
#22208=EDGE_CURVE('',#17205,#17204,#10088,.T.);
#22209=EDGE_CURVE('',#17206,#17205,#11439,.T.);
#22210=EDGE_CURVE('',#17207,#17206,#11440,.T.);
#22211=EDGE_CURVE('',#17208,#17207,#8301,.T.);
#22212=EDGE_CURVE('',#17209,#17208,#11441,.T.);
#22213=EDGE_CURVE('',#17210,#17209,#11442,.T.);
#22214=EDGE_CURVE('',#17211,#17210,#8302,.T.);
#22215=EDGE_CURVE('',#17212,#17211,#11443,.T.);
#22216=EDGE_CURVE('',#17213,#17212,#11444,.T.);
#22217=EDGE_CURVE('',#17214,#17213,#8303,.T.);
#22218=EDGE_CURVE('',#17215,#17214,#11445,.T.);
#22219=EDGE_CURVE('',#17216,#17215,#11446,.T.);
#22220=EDGE_CURVE('',#17217,#17216,#8304,.T.);
#22221=EDGE_CURVE('',#17218,#17217,#11447,.T.);
#22222=EDGE_CURVE('',#17219,#17218,#11448,.T.);
#22223=EDGE_CURVE('',#17220,#17219,#8305,.T.);
#22224=EDGE_CURVE('',#17221,#17220,#11449,.T.);
#22225=EDGE_CURVE('',#17222,#17221,#11450,.T.);
#22226=EDGE_CURVE('',#17223,#17222,#8306,.T.);
#22227=EDGE_CURVE('',#17224,#17223,#11451,.T.);
#22228=EDGE_CURVE('',#17189,#17224,#11452,.T.);
#22229=EDGE_CURVE('',#17225,#17225,#8307,.T.);
#22230=EDGE_CURVE('',#17226,#17227,#8308,.T.);
#22231=EDGE_CURVE('',#17227,#17223,#8309,.T.);
#22232=EDGE_CURVE('',#17223,#17226,#8310,.T.);
#22233=EDGE_CURVE('',#17228,#17229,#8311,.T.);
#22234=EDGE_CURVE('',#17229,#17227,#10089,.T.);
#22235=EDGE_CURVE('',#17226,#17228,#10090,.T.);
#22236=EDGE_CURVE('',#17230,#17222,#8312,.T.);
#22237=EDGE_CURVE('',#17221,#17231,#212,.F.);
#22238=EDGE_CURVE('',#17231,#17230,#11453,.T.);
#22239=EDGE_CURVE('',#17232,#17230,#8313,.T.);
#22240=EDGE_CURVE('',#17230,#17233,#10091,.T.);
#22241=EDGE_CURVE('',#17233,#17228,#8314,.T.);
#22242=EDGE_CURVE('',#17228,#17232,#10092,.T.);
#22243=EDGE_CURVE('',#17232,#17222,#8315,.T.);
#22244=EDGE_CURVE('',#17233,#17229,#8316,.T.);
#22245=EDGE_CURVE('',#17143,#17229,#11454,.T.);
#22246=EDGE_CURVE('',#17227,#17187,#11455,.T.);
#22247=EDGE_CURVE('',#17233,#17144,#11456,.T.);
#22248=EDGE_CURVE('',#17231,#17145,#11457,.T.);
#22249=EDGE_CURVE('',#17234,#17207,#8317,.T.);
#22250=EDGE_CURVE('',#17206,#17235,#213,.F.);
#22251=EDGE_CURVE('',#17235,#17234,#11458,.T.);
#22252=EDGE_CURVE('',#17236,#17234,#8318,.T.);
#22253=EDGE_CURVE('',#17234,#17237,#10093,.T.);
#22254=EDGE_CURVE('',#17237,#17238,#8319,.T.);
#22255=EDGE_CURVE('',#17238,#17236,#10094,.T.);
#22256=EDGE_CURVE('',#17236,#17207,#8320,.T.);
#22257=EDGE_CURVE('',#17239,#17237,#8321,.T.);
#22258=EDGE_CURVE('',#17237,#17123,#11459,.T.);
#22259=EDGE_CURVE('',#17158,#17239,#11460,.T.);
#22260=EDGE_CURVE('',#17239,#17238,#8322,.T.);
#22261=EDGE_CURVE('',#17236,#17240,#8323,.T.);
#22262=EDGE_CURVE('',#17208,#17240,#8324,.T.);
#22263=EDGE_CURVE('',#17240,#17238,#10095,.T.);
#22264=EDGE_CURVE('',#17239,#17241,#10096,.T.);
#22265=EDGE_CURVE('',#17241,#17240,#8325,.T.);
#22266=EDGE_CURVE('',#17242,#17157,#11461,.T.);
#22267=EDGE_CURVE('',#17241,#17242,#11462,.T.);
#22268=EDGE_CURVE('',#17243,#17147,#11463,.T.);
#22269=EDGE_CURVE('',#17146,#17244,#11464,.T.);
#22270=EDGE_CURVE('',#17244,#17245,#10097,.T.);
#22271=EDGE_CURVE('',#17245,#17243,#10098,.T.);
#22272=EDGE_CURVE('',#17244,#17246,#10099,.T.);
#22273=EDGE_CURVE('',#17246,#17247,#8326,.T.);
#22274=EDGE_CURVE('',#17247,#17245,#10100,.T.);
#22275=EDGE_CURVE('',#17220,#17246,#8327,.T.);
#22276=EDGE_CURVE('',#17246,#17231,#11465,.T.);
#22277=EDGE_CURVE('',#17220,#17247,#8328,.T.);
#22278=EDGE_CURVE('',#17243,#17248,#1830,.T.);
#22279=EDGE_CURVE('',#17249,#17248,#11466,.T.);
#22280=EDGE_CURVE('',#17249,#17148,#11467,.T.);
#22281=EDGE_CURVE('',#17250,#17247,#8329,.T.);
#22282=EDGE_CURVE('',#17248,#17250,#10101,.T.);
#22283=EDGE_CURVE('',#17250,#17219,#10102,.T.);
#22284=EDGE_CURVE('',#17232,#17226,#8330,.T.);
#22285=EDGE_CURVE('',#17187,#17224,#214,.F.);
#22286=EDGE_CURVE('',#17218,#17249,#215,.F.);
#22287=EDGE_CURVE('',#17242,#17251,#11468,.T.);
#22288=EDGE_CURVE('',#17251,#17210,#8331,.T.);
#22289=EDGE_CURVE('',#17209,#17242,#216,.T.);
#22290=EDGE_CURVE('',#17208,#17241,#8332,.T.);
#22291=EDGE_CURVE('',#17252,#17251,#8333,.T.);
#22292=EDGE_CURVE('',#17251,#17253,#10103,.T.);
#22293=EDGE_CURVE('',#17253,#17254,#8334,.T.);
#22294=EDGE_CURVE('',#17254,#17252,#10104,.T.);
#22295=EDGE_CURVE('',#17253,#17255,#8335,.T.);
#22296=EDGE_CURVE('',#17255,#17254,#8336,.T.);
#22297=EDGE_CURVE('',#17252,#17210,#8337,.T.);
#22298=EDGE_CURVE('',#17235,#17124,#11469,.T.);
#22299=EDGE_CURVE('',#17252,#17256,#8338,.T.);
#22300=EDGE_CURVE('',#17211,#17256,#8339,.T.);
#22301=EDGE_CURVE('',#17256,#17254,#10105,.T.);
#22302=EDGE_CURVE('',#17253,#17156,#11470,.T.);
#22303=EDGE_CURVE('',#17155,#17255,#11471,.T.);
#22304=EDGE_CURVE('',#17255,#17257,#10106,.T.);
#22305=EDGE_CURVE('',#17257,#17256,#8340,.T.);
#22306=EDGE_CURVE('',#17258,#17259,#11472,.T.);
#22307=EDGE_CURVE('',#17259,#17213,#8341,.T.);
#22308=EDGE_CURVE('',#17212,#17258,#217,.T.);
#22309=EDGE_CURVE('',#17211,#17257,#8342,.T.);
#22310=EDGE_CURVE('',#17257,#17258,#11473,.T.);
#22311=EDGE_CURVE('',#17260,#17261,#8343,.F.);
#22312=EDGE_CURVE('',#17262,#17260,#8344,.F.);
#22313=EDGE_CURVE('',#17261,#17262,#8345,.F.);
#22314=EDGE_CURVE('',#17152,#17262,#11474,.T.);
#22315=EDGE_CURVE('',#17260,#17153,#11475,.T.);
#22316=EDGE_CURVE('',#17262,#17263,#10107,.T.);
#22317=EDGE_CURVE('',#17263,#17264,#8346,.T.);
#22318=EDGE_CURVE('',#17264,#17261,#10108,.T.);
#22319=EDGE_CURVE('',#17261,#17265,#10109,.T.);
#22320=EDGE_CURVE('',#17265,#17259,#8347,.T.);
#22321=EDGE_CURVE('',#17259,#17260,#10110,.T.);
#22322=EDGE_CURVE('',#17266,#17267,#11476,.T.);
#22323=EDGE_CURVE('',#17267,#17216,#8348,.T.);
#22324=EDGE_CURVE('',#17215,#17266,#218,.T.);
#22325=EDGE_CURVE('',#17214,#17263,#8349,.T.);
#22326=EDGE_CURVE('',#17263,#17266,#11477,.T.);
#22327=EDGE_CURVE('',#17268,#17269,#8350,.F.);
#22328=EDGE_CURVE('',#17270,#17268,#8351,.F.);
#22329=EDGE_CURVE('',#17269,#17270,#8352,.F.);
#22330=EDGE_CURVE('',#17149,#17270,#11478,.T.);
#22331=EDGE_CURVE('',#17268,#17150,#11479,.T.);
#22332=EDGE_CURVE('',#17270,#17271,#10111,.T.);
#22333=EDGE_CURVE('',#17271,#17272,#8353,.T.);
#22334=EDGE_CURVE('',#17272,#17269,#10112,.T.);
#22335=EDGE_CURVE('',#17269,#17273,#10113,.T.);
#22336=EDGE_CURVE('',#17273,#17267,#8354,.T.);
#22337=EDGE_CURVE('',#17267,#17268,#10114,.T.);
#22338=EDGE_CURVE('',#17217,#17271,#8355,.T.);
#22339=EDGE_CURVE('',#17271,#17249,#11480,.T.);
#22340=EDGE_CURVE('',#17217,#17272,#8356,.T.);
#22341=EDGE_CURVE('',#17273,#17216,#8357,.T.);
#22342=EDGE_CURVE('',#17214,#17264,#8358,.T.);
#22343=EDGE_CURVE('',#17265,#17213,#8359,.T.);
#22344=EDGE_CURVE('',#17265,#17264,#8360,.T.);
#22345=EDGE_CURVE('',#17273,#17272,#8361,.T.);
#22346=EDGE_CURVE('',#17266,#17151,#11481,.T.);
#22347=EDGE_CURVE('',#17258,#17154,#11482,.T.);
#22348=EDGE_CURVE('',#17186,#17189,#8362,.T.);
#22349=EDGE_CURVE('',#17225,#17179,#8363,.T.);
#22350=EDGE_CURVE('',#17165,#17169,#8364,.T.);
#22351=EDGE_CURVE('',#17274,#17136,#11483,.T.);
#22352=EDGE_CURVE('',#17190,#17274,#219,.F.);
#22353=EDGE_CURVE('',#17275,#17276,#8365,.T.);
#22354=EDGE_CURVE('',#17276,#17277,#8366,.T.);
#22355=EDGE_CURVE('',#17277,#17275,#8367,.T.);
#22356=EDGE_CURVE('',#17275,#17135,#11484,.T.);
#22357=EDGE_CURVE('',#17134,#17276,#11485,.T.);
#22358=EDGE_CURVE('',#17278,#17275,#10115,.T.);
#22359=EDGE_CURVE('',#17274,#17278,#11486,.T.);
#22360=EDGE_CURVE('',#17277,#17279,#10116,.T.);
#22361=EDGE_CURVE('',#17278,#17279,#8368,.T.);
#22362=EDGE_CURVE('',#17276,#17280,#10117,.T.);
#22363=EDGE_CURVE('',#17281,#17280,#8369,.T.);
#22364=EDGE_CURVE('',#17281,#17277,#10118,.T.);
#22365=EDGE_CURVE('',#17192,#17280,#8370,.T.);
#22366=EDGE_CURVE('',#17280,#17282,#11487,.T.);
#22367=EDGE_CURVE('',#17282,#17193,#220,.F.);
#22368=EDGE_CURVE('',#17191,#17279,#8371,.T.);
#22369=EDGE_CURVE('',#17279,#17281,#8372,.T.);
#22370=EDGE_CURVE('',#17281,#17192,#8373,.T.);
#22371=EDGE_CURVE('',#17278,#17191,#8374,.T.);
#22372=EDGE_CURVE('',#17282,#17133,#11488,.T.);
#22373=EDGE_CURVE('',#17283,#17284,#8375,.T.);
#22374=EDGE_CURVE('',#17284,#17285,#8376,.T.);
#22375=EDGE_CURVE('',#17285,#17283,#8377,.T.);
#22376=EDGE_CURVE('',#17283,#17126,#11489,.T.);
#22377=EDGE_CURVE('',#17125,#17284,#11490,.T.);
#22378=EDGE_CURVE('',#17202,#17283,#10119,.T.);
#22379=EDGE_CURVE('',#17201,#17127,#11491,.T.);
#22380=EDGE_CURVE('',#17285,#17286,#10120,.T.);
#22381=EDGE_CURVE('',#17286,#17203,#10121,.T.);
#22382=EDGE_CURVE('',#17284,#17205,#10122,.T.);
#22383=EDGE_CURVE('',#17204,#17287,#10123,.T.);
#22384=EDGE_CURVE('',#17287,#17285,#10124,.T.);
#22385=EDGE_CURVE('',#17288,#17289,#8378,.T.);
#22386=EDGE_CURVE('',#17289,#17290,#8379,.T.);
#22387=EDGE_CURVE('',#17290,#17288,#8380,.T.);
#22388=EDGE_CURVE('',#17288,#17129,#11492,.T.);
#22389=EDGE_CURVE('',#17128,#17289,#11493,.T.);
#22390=EDGE_CURVE('',#17197,#17288,#10125,.T.);
#22391=EDGE_CURVE('',#17291,#17196,#221,.F.);
#22392=EDGE_CURVE('',#17291,#17130,#11494,.T.);
#22393=EDGE_CURVE('',#17290,#17292,#10126,.T.);
#22394=EDGE_CURVE('',#17292,#17198,#10127,.T.);
#22395=EDGE_CURVE('',#17289,#17200,#10128,.T.);
#22396=EDGE_CURVE('',#17199,#17293,#10129,.T.);
#22397=EDGE_CURVE('',#17293,#17290,#10130,.T.);
#22398=EDGE_CURVE('',#17294,#17295,#8381,.T.);
#22399=EDGE_CURVE('',#17295,#17296,#8382,.T.);
#22400=EDGE_CURVE('',#17296,#17294,#8383,.T.);
#22401=EDGE_CURVE('',#17294,#17132,#11495,.T.);
#22402=EDGE_CURVE('',#17131,#17295,#11496,.T.);
#22403=EDGE_CURVE('',#17297,#17294,#10131,.T.);
#22404=EDGE_CURVE('',#17282,#17297,#11497,.T.);
#22405=EDGE_CURVE('',#17296,#17298,#10132,.T.);
#22406=EDGE_CURVE('',#17297,#17298,#8384,.T.);
#22407=EDGE_CURVE('',#17295,#17299,#10133,.T.);
#22408=EDGE_CURVE('',#17300,#17299,#8385,.T.);
#22409=EDGE_CURVE('',#17300,#17296,#10134,.T.);
#22410=EDGE_CURVE('',#17195,#17299,#8386,.T.);
#22411=EDGE_CURVE('',#17299,#17291,#11498,.T.);
#22412=EDGE_CURVE('',#17194,#17298,#8387,.T.);
#22413=EDGE_CURVE('',#17298,#17300,#8388,.T.);
#22414=EDGE_CURVE('',#17300,#17195,#8389,.T.);
#22415=EDGE_CURVE('',#17297,#17194,#8390,.T.);
#22416=EDGE_CURVE('',#17292,#17293,#8391,.T.);
#22417=EDGE_CURVE('',#17286,#17287,#8392,.T.);
#31161=ORIENTED_EDGE('',*,*,#22092,.T.);
#31162=ORIENTED_EDGE('',*,*,#22093,.T.);
#31163=ORIENTED_EDGE('',*,*,#22094,.T.);
#31164=ORIENTED_EDGE('',*,*,#22095,.T.);
#31165=ORIENTED_EDGE('',*,*,#22096,.T.);
#31166=ORIENTED_EDGE('',*,*,#22094,.F.);
#31167=ORIENTED_EDGE('',*,*,#22096,.F.);
#31168=ORIENTED_EDGE('',*,*,#22097,.T.);
#31169=ORIENTED_EDGE('',*,*,#22098,.F.);
#31170=ORIENTED_EDGE('',*,*,#22099,.F.);
#31171=ORIENTED_EDGE('',*,*,#22097,.F.);
#31172=ORIENTED_EDGE('',*,*,#22095,.F.);
#31173=ORIENTED_EDGE('',*,*,#22100,.F.);
#31174=ORIENTED_EDGE('',*,*,#22101,.T.);
#31175=ORIENTED_EDGE('',*,*,#22092,.F.);
#31176=ORIENTED_EDGE('',*,*,#22093,.F.);
#31177=ORIENTED_EDGE('',*,*,#22101,.F.);
#31178=ORIENTED_EDGE('',*,*,#22102,.F.);
#31179=ORIENTED_EDGE('',*,*,#22098,.T.);
#31180=ORIENTED_EDGE('',*,*,#22099,.T.);
#31181=ORIENTED_EDGE('',*,*,#22103,.T.);
#31182=ORIENTED_EDGE('',*,*,#22104,.T.);
#31183=ORIENTED_EDGE('',*,*,#22103,.F.);
#31184=ORIENTED_EDGE('',*,*,#22104,.F.);
#31185=ORIENTED_EDGE('',*,*,#22105,.T.);
#31186=ORIENTED_EDGE('',*,*,#22106,.T.);
#31187=ORIENTED_EDGE('',*,*,#22107,.F.);
#31188=ORIENTED_EDGE('',*,*,#22108,.T.);
#31189=ORIENTED_EDGE('',*,*,#22109,.T.);
#31190=ORIENTED_EDGE('',*,*,#22110,.F.);
#31191=ORIENTED_EDGE('',*,*,#22111,.T.);
#31192=ORIENTED_EDGE('',*,*,#22112,.T.);
#31193=ORIENTED_EDGE('',*,*,#22113,.F.);
#31194=ORIENTED_EDGE('',*,*,#22114,.T.);
#31195=ORIENTED_EDGE('',*,*,#22115,.T.);
#31196=ORIENTED_EDGE('',*,*,#22116,.F.);
#31197=ORIENTED_EDGE('',*,*,#22117,.T.);
#31198=ORIENTED_EDGE('',*,*,#22118,.T.);
#31199=ORIENTED_EDGE('',*,*,#22119,.F.);
#31200=ORIENTED_EDGE('',*,*,#22120,.T.);
#31201=ORIENTED_EDGE('',*,*,#22121,.T.);
#31202=ORIENTED_EDGE('',*,*,#22122,.F.);
#31203=ORIENTED_EDGE('',*,*,#22123,.T.);
#31204=ORIENTED_EDGE('',*,*,#22124,.T.);
#31205=ORIENTED_EDGE('',*,*,#22125,.F.);
#31206=ORIENTED_EDGE('',*,*,#22126,.T.);
#31207=ORIENTED_EDGE('',*,*,#22127,.T.);
#31208=ORIENTED_EDGE('',*,*,#22128,.F.);
#31209=ORIENTED_EDGE('',*,*,#22129,.T.);
#31210=ORIENTED_EDGE('',*,*,#22130,.T.);
#31211=ORIENTED_EDGE('',*,*,#22131,.F.);
#31212=ORIENTED_EDGE('',*,*,#22132,.T.);
#31213=ORIENTED_EDGE('',*,*,#22133,.T.);
#31214=ORIENTED_EDGE('',*,*,#22134,.F.);
#31215=ORIENTED_EDGE('',*,*,#22135,.T.);
#31216=ORIENTED_EDGE('',*,*,#22136,.T.);
#31217=ORIENTED_EDGE('',*,*,#22137,.F.);
#31218=ORIENTED_EDGE('',*,*,#22138,.T.);
#31219=ORIENTED_EDGE('',*,*,#22139,.T.);
#31220=ORIENTED_EDGE('',*,*,#22140,.F.);
#31221=ORIENTED_EDGE('',*,*,#22141,.T.);
#31222=ORIENTED_EDGE('',*,*,#22142,.T.);
#31223=ORIENTED_EDGE('',*,*,#22143,.T.);
#31224=ORIENTED_EDGE('',*,*,#22141,.F.);
#31225=ORIENTED_EDGE('',*,*,#22144,.T.);
#31226=ORIENTED_EDGE('',*,*,#22119,.T.);
#31227=ORIENTED_EDGE('',*,*,#22145,.T.);
#31228=ORIENTED_EDGE('',*,*,#22144,.F.);
#31229=ORIENTED_EDGE('',*,*,#22146,.F.);
#31230=ORIENTED_EDGE('',*,*,#22147,.T.);
#31231=ORIENTED_EDGE('',*,*,#22148,.F.);
#31232=ORIENTED_EDGE('',*,*,#22149,.T.);
#31233=ORIENTED_EDGE('',*,*,#22120,.F.);
#31234=ORIENTED_EDGE('',*,*,#22143,.F.);
#31235=ORIENTED_EDGE('',*,*,#22150,.T.);
#31236=ORIENTED_EDGE('',*,*,#22151,.T.);
#31237=ORIENTED_EDGE('',*,*,#22152,.T.);
#31238=ORIENTED_EDGE('',*,*,#22146,.T.);
#31239=ORIENTED_EDGE('',*,*,#22142,.F.);
#31240=ORIENTED_EDGE('',*,*,#22153,.T.);
#31241=ORIENTED_EDGE('',*,*,#22154,.T.);
#31242=ORIENTED_EDGE('',*,*,#22155,.T.);
#31243=ORIENTED_EDGE('',*,*,#22156,.T.);
#31244=ORIENTED_EDGE('',*,*,#22157,.T.);
#31245=ORIENTED_EDGE('',*,*,#22158,.T.);
#31246=ORIENTED_EDGE('',*,*,#22102,.T.);
#31247=ORIENTED_EDGE('',*,*,#22100,.T.);
#31248=ORIENTED_EDGE('',*,*,#22158,.F.);
#31249=ORIENTED_EDGE('',*,*,#22157,.F.);
#31250=ORIENTED_EDGE('',*,*,#22159,.F.);
#31251=ORIENTED_EDGE('',*,*,#22160,.T.);
#31252=ORIENTED_EDGE('',*,*,#22161,.T.);
#31253=ORIENTED_EDGE('',*,*,#22162,.T.);
#31254=ORIENTED_EDGE('',*,*,#22159,.T.);
#31255=ORIENTED_EDGE('',*,*,#22162,.F.);
#31256=ORIENTED_EDGE('',*,*,#22160,.F.);
#31257=ORIENTED_EDGE('',*,*,#22161,.F.);
#31258=ORIENTED_EDGE('',*,*,#22163,.T.);
#31259=ORIENTED_EDGE('',*,*,#22164,.F.);
#31260=ORIENTED_EDGE('',*,*,#22165,.F.);
#31261=ORIENTED_EDGE('',*,*,#22163,.F.);
#31262=ORIENTED_EDGE('',*,*,#22166,.T.);
#31263=ORIENTED_EDGE('',*,*,#22167,.T.);
#31264=ORIENTED_EDGE('',*,*,#22168,.T.);
#31265=ORIENTED_EDGE('',*,*,#22164,.T.);
#31266=ORIENTED_EDGE('',*,*,#22165,.T.);
#31267=ORIENTED_EDGE('',*,*,#22168,.F.);
#31268=ORIENTED_EDGE('',*,*,#22169,.F.);
#31269=ORIENTED_EDGE('',*,*,#22170,.T.);
#31270=ORIENTED_EDGE('',*,*,#22166,.F.);
#31271=ORIENTED_EDGE('',*,*,#22167,.F.);
#31272=ORIENTED_EDGE('',*,*,#22170,.F.);
#31273=ORIENTED_EDGE('',*,*,#22171,.F.);
#31274=ORIENTED_EDGE('',*,*,#22172,.T.);
#31275=ORIENTED_EDGE('',*,*,#22173,.T.);
#31276=ORIENTED_EDGE('',*,*,#22122,.T.);
#31277=ORIENTED_EDGE('',*,*,#22174,.T.);
#31278=ORIENTED_EDGE('',*,*,#22175,.T.);
#31279=ORIENTED_EDGE('',*,*,#22176,.T.);
#31280=ORIENTED_EDGE('',*,*,#22177,.T.);
#31281=ORIENTED_EDGE('',*,*,#22178,.T.);
#31282=ORIENTED_EDGE('',*,*,#22179,.T.);
#31283=ORIENTED_EDGE('',*,*,#22180,.T.);
#31284=ORIENTED_EDGE('',*,*,#22148,.T.);
#31285=ORIENTED_EDGE('',*,*,#22181,.T.);
#31286=ORIENTED_EDGE('',*,*,#22179,.F.);
#31287=ORIENTED_EDGE('',*,*,#22182,.T.);
#31288=ORIENTED_EDGE('',*,*,#22177,.F.);
#31289=ORIENTED_EDGE('',*,*,#22175,.F.);
#31290=ORIENTED_EDGE('',*,*,#22183,.T.);
#31291=ORIENTED_EDGE('',*,*,#22172,.F.);
#31292=ORIENTED_EDGE('',*,*,#22173,.F.);
#31293=ORIENTED_EDGE('',*,*,#22184,.F.);
#31294=ORIENTED_EDGE('',*,*,#22185,.F.);
#31295=ORIENTED_EDGE('',*,*,#22186,.T.);
#31296=ORIENTED_EDGE('',*,*,#22123,.F.);
#31297=ORIENTED_EDGE('',*,*,#22183,.F.);
#31298=ORIENTED_EDGE('',*,*,#22187,.T.);
#31299=ORIENTED_EDGE('',*,*,#22188,.F.);
#31300=ORIENTED_EDGE('',*,*,#22184,.T.);
#31301=ORIENTED_EDGE('',*,*,#22178,.F.);
#31302=ORIENTED_EDGE('',*,*,#22189,.F.);
#31303=ORIENTED_EDGE('',*,*,#22187,.F.);
#31304=ORIENTED_EDGE('',*,*,#22182,.F.);
#31305=ORIENTED_EDGE('',*,*,#22190,.T.);
#31306=ORIENTED_EDGE('',*,*,#22191,.T.);
#31307=ORIENTED_EDGE('',*,*,#22189,.T.);
#31308=ORIENTED_EDGE('',*,*,#22181,.F.);
#31309=ORIENTED_EDGE('',*,*,#22147,.F.);
#31310=ORIENTED_EDGE('',*,*,#22152,.F.);
#31311=ORIENTED_EDGE('',*,*,#22192,.F.);
#31312=ORIENTED_EDGE('',*,*,#22154,.F.);
#31313=ORIENTED_EDGE('',*,*,#22193,.F.);
#31314=ORIENTED_EDGE('',*,*,#22194,.F.);
#31315=ORIENTED_EDGE('',*,*,#22195,.F.);
#31316=ORIENTED_EDGE('',*,*,#22196,.F.);
#31317=ORIENTED_EDGE('',*,*,#22197,.F.);
#31318=ORIENTED_EDGE('',*,*,#22198,.F.);
#31319=ORIENTED_EDGE('',*,*,#22199,.F.);
#31320=ORIENTED_EDGE('',*,*,#22200,.F.);
#31321=ORIENTED_EDGE('',*,*,#22201,.F.);
#31322=ORIENTED_EDGE('',*,*,#22202,.F.);
#31323=ORIENTED_EDGE('',*,*,#22203,.F.);
#31324=ORIENTED_EDGE('',*,*,#22204,.F.);
#31325=ORIENTED_EDGE('',*,*,#22205,.F.);
#31326=ORIENTED_EDGE('',*,*,#22206,.F.);
#31327=ORIENTED_EDGE('',*,*,#22207,.F.);
#31328=ORIENTED_EDGE('',*,*,#22208,.F.);
#31329=ORIENTED_EDGE('',*,*,#22209,.F.);
#31330=ORIENTED_EDGE('',*,*,#22210,.F.);
#31331=ORIENTED_EDGE('',*,*,#22211,.F.);
#31332=ORIENTED_EDGE('',*,*,#22212,.F.);
#31333=ORIENTED_EDGE('',*,*,#22213,.F.);
#31334=ORIENTED_EDGE('',*,*,#22214,.F.);
#31335=ORIENTED_EDGE('',*,*,#22215,.F.);
#31336=ORIENTED_EDGE('',*,*,#22216,.F.);
#31337=ORIENTED_EDGE('',*,*,#22217,.F.);
#31338=ORIENTED_EDGE('',*,*,#22218,.F.);
#31339=ORIENTED_EDGE('',*,*,#22219,.F.);
#31340=ORIENTED_EDGE('',*,*,#22220,.F.);
#31341=ORIENTED_EDGE('',*,*,#22221,.F.);
#31342=ORIENTED_EDGE('',*,*,#22222,.F.);
#31343=ORIENTED_EDGE('',*,*,#22223,.F.);
#31344=ORIENTED_EDGE('',*,*,#22224,.F.);
#31345=ORIENTED_EDGE('',*,*,#22225,.F.);
#31346=ORIENTED_EDGE('',*,*,#22226,.F.);
#31347=ORIENTED_EDGE('',*,*,#22227,.F.);
#31348=ORIENTED_EDGE('',*,*,#22228,.F.);
#31349=ORIENTED_EDGE('',*,*,#22190,.F.);
#31350=ORIENTED_EDGE('',*,*,#22229,.F.);
#31351=ORIENTED_EDGE('',*,*,#22230,.T.);
#31352=ORIENTED_EDGE('',*,*,#22231,.T.);
#31353=ORIENTED_EDGE('',*,*,#22232,.T.);
#31354=ORIENTED_EDGE('',*,*,#22233,.T.);
#31355=ORIENTED_EDGE('',*,*,#22234,.T.);
#31356=ORIENTED_EDGE('',*,*,#22230,.F.);
#31357=ORIENTED_EDGE('',*,*,#22235,.T.);
#31358=ORIENTED_EDGE('',*,*,#22236,.T.);
#31359=ORIENTED_EDGE('',*,*,#22225,.T.);
#31360=ORIENTED_EDGE('',*,*,#22237,.T.);
#31361=ORIENTED_EDGE('',*,*,#22238,.T.);
#31362=ORIENTED_EDGE('',*,*,#22239,.T.);
#31363=ORIENTED_EDGE('',*,*,#22240,.T.);
#31364=ORIENTED_EDGE('',*,*,#22241,.T.);
#31365=ORIENTED_EDGE('',*,*,#22242,.T.);
#31366=ORIENTED_EDGE('',*,*,#22239,.F.);
#31367=ORIENTED_EDGE('',*,*,#22243,.T.);
#31368=ORIENTED_EDGE('',*,*,#22236,.F.);
#31369=ORIENTED_EDGE('',*,*,#22241,.F.);
#31370=ORIENTED_EDGE('',*,*,#22244,.T.);
#31371=ORIENTED_EDGE('',*,*,#22233,.F.);
#31372=ORIENTED_EDGE('',*,*,#22234,.F.);
#31373=ORIENTED_EDGE('',*,*,#22245,.F.);
#31374=ORIENTED_EDGE('',*,*,#22124,.F.);
#31375=ORIENTED_EDGE('',*,*,#22186,.F.);
#31376=ORIENTED_EDGE('',*,*,#22246,.F.);
#31377=ORIENTED_EDGE('',*,*,#22244,.F.);
#31378=ORIENTED_EDGE('',*,*,#22247,.T.);
#31379=ORIENTED_EDGE('',*,*,#22125,.T.);
#31380=ORIENTED_EDGE('',*,*,#22245,.T.);
#31381=ORIENTED_EDGE('',*,*,#22240,.F.);
#31382=ORIENTED_EDGE('',*,*,#22238,.F.);
#31383=ORIENTED_EDGE('',*,*,#22248,.T.);
#31384=ORIENTED_EDGE('',*,*,#22126,.F.);
#31385=ORIENTED_EDGE('',*,*,#22247,.F.);
#31386=ORIENTED_EDGE('',*,*,#22249,.T.);
#31387=ORIENTED_EDGE('',*,*,#22210,.T.);
#31388=ORIENTED_EDGE('',*,*,#22250,.T.);
#31389=ORIENTED_EDGE('',*,*,#22251,.T.);
#31390=ORIENTED_EDGE('',*,*,#22252,.T.);
#31391=ORIENTED_EDGE('',*,*,#22253,.T.);
#31392=ORIENTED_EDGE('',*,*,#22254,.T.);
#31393=ORIENTED_EDGE('',*,*,#22255,.T.);
#31394=ORIENTED_EDGE('',*,*,#22252,.F.);
#31395=ORIENTED_EDGE('',*,*,#22256,.T.);
#31396=ORIENTED_EDGE('',*,*,#22249,.F.);
#31397=ORIENTED_EDGE('',*,*,#22257,.T.);
#31398=ORIENTED_EDGE('',*,*,#22258,.T.);
#31399=ORIENTED_EDGE('',*,*,#22140,.T.);
#31400=ORIENTED_EDGE('',*,*,#22259,.T.);
#31401=ORIENTED_EDGE('',*,*,#22257,.F.);
#31402=ORIENTED_EDGE('',*,*,#22260,.T.);
#31403=ORIENTED_EDGE('',*,*,#22254,.F.);
#31404=ORIENTED_EDGE('',*,*,#22256,.F.);
#31405=ORIENTED_EDGE('',*,*,#22261,.T.);
#31406=ORIENTED_EDGE('',*,*,#22262,.F.);
#31407=ORIENTED_EDGE('',*,*,#22211,.T.);
#31408=ORIENTED_EDGE('',*,*,#22255,.F.);
#31409=ORIENTED_EDGE('',*,*,#22263,.F.);
#31410=ORIENTED_EDGE('',*,*,#22261,.F.);
#31411=ORIENTED_EDGE('',*,*,#22260,.F.);
#31412=ORIENTED_EDGE('',*,*,#22264,.T.);
#31413=ORIENTED_EDGE('',*,*,#22265,.T.);
#31414=ORIENTED_EDGE('',*,*,#22263,.T.);
#31415=ORIENTED_EDGE('',*,*,#22259,.F.);
#31416=ORIENTED_EDGE('',*,*,#22139,.F.);
#31417=ORIENTED_EDGE('',*,*,#22266,.F.);
#31418=ORIENTED_EDGE('',*,*,#22267,.F.);
#31419=ORIENTED_EDGE('',*,*,#22264,.F.);
#31420=ORIENTED_EDGE('',*,*,#22268,.T.);
#31421=ORIENTED_EDGE('',*,*,#22128,.T.);
#31422=ORIENTED_EDGE('',*,*,#22269,.T.);
#31423=ORIENTED_EDGE('',*,*,#22270,.T.);
#31424=ORIENTED_EDGE('',*,*,#22271,.T.);
#31425=ORIENTED_EDGE('',*,*,#22272,.T.);
#31426=ORIENTED_EDGE('',*,*,#22273,.T.);
#31427=ORIENTED_EDGE('',*,*,#22274,.T.);
#31428=ORIENTED_EDGE('',*,*,#22270,.F.);
#31429=ORIENTED_EDGE('',*,*,#22275,.T.);
#31430=ORIENTED_EDGE('',*,*,#22276,.T.);
#31431=ORIENTED_EDGE('',*,*,#22237,.F.);
#31432=ORIENTED_EDGE('',*,*,#22224,.T.);
#31433=ORIENTED_EDGE('',*,*,#22275,.F.);
#31434=ORIENTED_EDGE('',*,*,#22277,.T.);
#31435=ORIENTED_EDGE('',*,*,#22273,.F.);
#31436=ORIENTED_EDGE('',*,*,#22268,.F.);
#31437=ORIENTED_EDGE('',*,*,#22278,.T.);
#31438=ORIENTED_EDGE('',*,*,#22279,.F.);
#31439=ORIENTED_EDGE('',*,*,#22280,.T.);
#31440=ORIENTED_EDGE('',*,*,#22129,.F.);
#31441=ORIENTED_EDGE('',*,*,#22271,.F.);
#31442=ORIENTED_EDGE('',*,*,#22274,.F.);
#31443=ORIENTED_EDGE('',*,*,#22281,.F.);
#31444=ORIENTED_EDGE('',*,*,#22282,.F.);
#31445=ORIENTED_EDGE('',*,*,#22278,.F.);
#31446=ORIENTED_EDGE('',*,*,#22277,.F.);
#31447=ORIENTED_EDGE('',*,*,#22223,.T.);
#31448=ORIENTED_EDGE('',*,*,#22283,.F.);
#31449=ORIENTED_EDGE('',*,*,#22281,.T.);
#31450=ORIENTED_EDGE('',*,*,#22235,.F.);
#31451=ORIENTED_EDGE('',*,*,#22284,.F.);
#31452=ORIENTED_EDGE('',*,*,#22242,.F.);
#31453=ORIENTED_EDGE('',*,*,#22231,.F.);
#31454=ORIENTED_EDGE('',*,*,#22246,.T.);
#31455=ORIENTED_EDGE('',*,*,#22285,.T.);
#31456=ORIENTED_EDGE('',*,*,#22227,.T.);
#31457=ORIENTED_EDGE('',*,*,#22232,.F.);
#31458=ORIENTED_EDGE('',*,*,#22226,.T.);
#31459=ORIENTED_EDGE('',*,*,#22243,.F.);
#31460=ORIENTED_EDGE('',*,*,#22284,.T.);
#31461=ORIENTED_EDGE('',*,*,#22222,.T.);
#31462=ORIENTED_EDGE('',*,*,#22286,.T.);
#31463=ORIENTED_EDGE('',*,*,#22279,.T.);
#31464=ORIENTED_EDGE('',*,*,#22282,.T.);
#31465=ORIENTED_EDGE('',*,*,#22283,.T.);
#31466=ORIENTED_EDGE('',*,*,#22269,.F.);
#31467=ORIENTED_EDGE('',*,*,#22127,.F.);
#31468=ORIENTED_EDGE('',*,*,#22248,.F.);
#31469=ORIENTED_EDGE('',*,*,#22276,.F.);
#31470=ORIENTED_EDGE('',*,*,#22272,.F.);
#31471=ORIENTED_EDGE('',*,*,#22287,.T.);
#31472=ORIENTED_EDGE('',*,*,#22288,.T.);
#31473=ORIENTED_EDGE('',*,*,#22213,.T.);
#31474=ORIENTED_EDGE('',*,*,#22289,.T.);
#31475=ORIENTED_EDGE('',*,*,#22212,.T.);
#31476=ORIENTED_EDGE('',*,*,#22290,.T.);
#31477=ORIENTED_EDGE('',*,*,#22267,.T.);
#31478=ORIENTED_EDGE('',*,*,#22289,.F.);
#31479=ORIENTED_EDGE('',*,*,#22291,.T.);
#31480=ORIENTED_EDGE('',*,*,#22292,.T.);
#31481=ORIENTED_EDGE('',*,*,#22293,.T.);
#31482=ORIENTED_EDGE('',*,*,#22294,.T.);
#31483=ORIENTED_EDGE('',*,*,#22293,.F.);
#31484=ORIENTED_EDGE('',*,*,#22295,.T.);
#31485=ORIENTED_EDGE('',*,*,#22296,.T.);
#31486=ORIENTED_EDGE('',*,*,#22291,.F.);
#31487=ORIENTED_EDGE('',*,*,#22297,.T.);
#31488=ORIENTED_EDGE('',*,*,#22288,.F.);
#31489=ORIENTED_EDGE('',*,*,#22290,.F.);
#31490=ORIENTED_EDGE('',*,*,#22262,.T.);
#31491=ORIENTED_EDGE('',*,*,#22265,.F.);
#31492=ORIENTED_EDGE('',*,*,#22251,.F.);
#31493=ORIENTED_EDGE('',*,*,#22298,.T.);
#31494=ORIENTED_EDGE('',*,*,#22105,.F.);
#31495=ORIENTED_EDGE('',*,*,#22258,.F.);
#31496=ORIENTED_EDGE('',*,*,#22253,.F.);
#31497=ORIENTED_EDGE('',*,*,#22297,.F.);
#31498=ORIENTED_EDGE('',*,*,#22299,.T.);
#31499=ORIENTED_EDGE('',*,*,#22300,.F.);
#31500=ORIENTED_EDGE('',*,*,#22214,.T.);
#31501=ORIENTED_EDGE('',*,*,#22294,.F.);
#31502=ORIENTED_EDGE('',*,*,#22301,.F.);
#31503=ORIENTED_EDGE('',*,*,#22299,.F.);
#31504=ORIENTED_EDGE('',*,*,#22295,.F.);
#31505=ORIENTED_EDGE('',*,*,#22302,.T.);
#31506=ORIENTED_EDGE('',*,*,#22137,.T.);
#31507=ORIENTED_EDGE('',*,*,#22303,.T.);
#31508=ORIENTED_EDGE('',*,*,#22296,.F.);
#31509=ORIENTED_EDGE('',*,*,#22304,.T.);
#31510=ORIENTED_EDGE('',*,*,#22305,.T.);
#31511=ORIENTED_EDGE('',*,*,#22301,.T.);
#31512=ORIENTED_EDGE('',*,*,#22306,.T.);
#31513=ORIENTED_EDGE('',*,*,#22307,.T.);
#31514=ORIENTED_EDGE('',*,*,#22216,.T.);
#31515=ORIENTED_EDGE('',*,*,#22308,.T.);
#31516=ORIENTED_EDGE('',*,*,#22215,.T.);
#31517=ORIENTED_EDGE('',*,*,#22309,.T.);
#31518=ORIENTED_EDGE('',*,*,#22310,.T.);
#31519=ORIENTED_EDGE('',*,*,#22308,.F.);
#31520=ORIENTED_EDGE('',*,*,#22311,.F.);
#31521=ORIENTED_EDGE('',*,*,#22312,.F.);
#31522=ORIENTED_EDGE('',*,*,#22313,.F.);
#31523=ORIENTED_EDGE('',*,*,#22134,.T.);
#31524=ORIENTED_EDGE('',*,*,#22314,.T.);
#31525=ORIENTED_EDGE('',*,*,#22312,.T.);
#31526=ORIENTED_EDGE('',*,*,#22315,.T.);
#31527=ORIENTED_EDGE('',*,*,#22313,.T.);
#31528=ORIENTED_EDGE('',*,*,#22316,.T.);
#31529=ORIENTED_EDGE('',*,*,#22317,.T.);
#31530=ORIENTED_EDGE('',*,*,#22318,.T.);
#31531=ORIENTED_EDGE('',*,*,#22311,.T.);
#31532=ORIENTED_EDGE('',*,*,#22319,.T.);
#31533=ORIENTED_EDGE('',*,*,#22320,.T.);
#31534=ORIENTED_EDGE('',*,*,#22321,.T.);
#31535=ORIENTED_EDGE('',*,*,#22322,.T.);
#31536=ORIENTED_EDGE('',*,*,#22323,.T.);
#31537=ORIENTED_EDGE('',*,*,#22219,.T.);
#31538=ORIENTED_EDGE('',*,*,#22324,.T.);
#31539=ORIENTED_EDGE('',*,*,#22218,.T.);
#31540=ORIENTED_EDGE('',*,*,#22325,.T.);
#31541=ORIENTED_EDGE('',*,*,#22326,.T.);
#31542=ORIENTED_EDGE('',*,*,#22324,.F.);
#31543=ORIENTED_EDGE('',*,*,#22327,.F.);
#31544=ORIENTED_EDGE('',*,*,#22328,.F.);
#31545=ORIENTED_EDGE('',*,*,#22329,.F.);
#31546=ORIENTED_EDGE('',*,*,#22131,.T.);
#31547=ORIENTED_EDGE('',*,*,#22330,.T.);
#31548=ORIENTED_EDGE('',*,*,#22328,.T.);
#31549=ORIENTED_EDGE('',*,*,#22331,.T.);
#31550=ORIENTED_EDGE('',*,*,#22329,.T.);
#31551=ORIENTED_EDGE('',*,*,#22332,.T.);
#31552=ORIENTED_EDGE('',*,*,#22333,.T.);
#31553=ORIENTED_EDGE('',*,*,#22334,.T.);
#31554=ORIENTED_EDGE('',*,*,#22327,.T.);
#31555=ORIENTED_EDGE('',*,*,#22335,.T.);
#31556=ORIENTED_EDGE('',*,*,#22336,.T.);
#31557=ORIENTED_EDGE('',*,*,#22337,.T.);
#31558=ORIENTED_EDGE('',*,*,#22338,.T.);
#31559=ORIENTED_EDGE('',*,*,#22339,.T.);
#31560=ORIENTED_EDGE('',*,*,#22286,.F.);
#31561=ORIENTED_EDGE('',*,*,#22221,.T.);
#31562=ORIENTED_EDGE('',*,*,#22338,.F.);
#31563=ORIENTED_EDGE('',*,*,#22340,.T.);
#31564=ORIENTED_EDGE('',*,*,#22333,.F.);
#31565=ORIENTED_EDGE('',*,*,#22336,.F.);
#31566=ORIENTED_EDGE('',*,*,#22341,.T.);
#31567=ORIENTED_EDGE('',*,*,#22323,.F.);
#31568=ORIENTED_EDGE('',*,*,#22325,.F.);
#31569=ORIENTED_EDGE('',*,*,#22342,.T.);
#31570=ORIENTED_EDGE('',*,*,#22317,.F.);
#31571=ORIENTED_EDGE('',*,*,#22320,.F.);
#31572=ORIENTED_EDGE('',*,*,#22343,.T.);
#31573=ORIENTED_EDGE('',*,*,#22307,.F.);
#31574=ORIENTED_EDGE('',*,*,#22309,.F.);
#31575=ORIENTED_EDGE('',*,*,#22300,.T.);
#31576=ORIENTED_EDGE('',*,*,#22305,.F.);
#31577=ORIENTED_EDGE('',*,*,#22287,.F.);
#31578=ORIENTED_EDGE('',*,*,#22266,.T.);
#31579=ORIENTED_EDGE('',*,*,#22138,.F.);
#31580=ORIENTED_EDGE('',*,*,#22302,.F.);
#31581=ORIENTED_EDGE('',*,*,#22292,.F.);
#31582=ORIENTED_EDGE('',*,*,#22319,.F.);
#31583=ORIENTED_EDGE('',*,*,#22318,.F.);
#31584=ORIENTED_EDGE('',*,*,#22344,.F.);
#31585=ORIENTED_EDGE('',*,*,#22343,.F.);
#31586=ORIENTED_EDGE('',*,*,#22344,.T.);
#31587=ORIENTED_EDGE('',*,*,#22342,.F.);
#31588=ORIENTED_EDGE('',*,*,#22217,.T.);
#31589=ORIENTED_EDGE('',*,*,#22335,.F.);
#31590=ORIENTED_EDGE('',*,*,#22334,.F.);
#31591=ORIENTED_EDGE('',*,*,#22345,.F.);
#31592=ORIENTED_EDGE('',*,*,#22341,.F.);
#31593=ORIENTED_EDGE('',*,*,#22345,.T.);
#31594=ORIENTED_EDGE('',*,*,#22340,.F.);
#31595=ORIENTED_EDGE('',*,*,#22220,.T.);
#31596=ORIENTED_EDGE('',*,*,#22330,.F.);
#31597=ORIENTED_EDGE('',*,*,#22130,.F.);
#31598=ORIENTED_EDGE('',*,*,#22280,.F.);
#31599=ORIENTED_EDGE('',*,*,#22339,.F.);
#31600=ORIENTED_EDGE('',*,*,#22332,.F.);
#31601=ORIENTED_EDGE('',*,*,#22314,.F.);
#31602=ORIENTED_EDGE('',*,*,#22133,.F.);
#31603=ORIENTED_EDGE('',*,*,#22346,.F.);
#31604=ORIENTED_EDGE('',*,*,#22326,.F.);
#31605=ORIENTED_EDGE('',*,*,#22316,.F.);
#31606=ORIENTED_EDGE('',*,*,#22303,.F.);
#31607=ORIENTED_EDGE('',*,*,#22136,.F.);
#31608=ORIENTED_EDGE('',*,*,#22347,.F.);
#31609=ORIENTED_EDGE('',*,*,#22310,.F.);
#31610=ORIENTED_EDGE('',*,*,#22304,.F.);
#31611=ORIENTED_EDGE('',*,*,#22348,.T.);
#31612=ORIENTED_EDGE('',*,*,#22228,.T.);
#31613=ORIENTED_EDGE('',*,*,#22285,.F.);
#31614=ORIENTED_EDGE('',*,*,#22185,.T.);
#31615=ORIENTED_EDGE('',*,*,#22348,.F.);
#31616=ORIENTED_EDGE('',*,*,#22188,.T.);
#31617=ORIENTED_EDGE('',*,*,#22191,.F.);
#31618=ORIENTED_EDGE('',*,*,#22229,.T.);
#31619=ORIENTED_EDGE('',*,*,#22349,.T.);
#31620=ORIENTED_EDGE('',*,*,#22171,.T.);
#31621=ORIENTED_EDGE('',*,*,#22169,.T.);
#31622=ORIENTED_EDGE('',*,*,#22349,.F.);
#31623=ORIENTED_EDGE('',*,*,#22192,.T.);
#31624=ORIENTED_EDGE('',*,*,#22151,.F.);
#31625=ORIENTED_EDGE('',*,*,#22350,.T.);
#31626=ORIENTED_EDGE('',*,*,#22155,.F.);
#31627=ORIENTED_EDGE('',*,*,#22145,.F.);
#31628=ORIENTED_EDGE('',*,*,#22118,.F.);
#31629=ORIENTED_EDGE('',*,*,#22351,.F.);
#31630=ORIENTED_EDGE('',*,*,#22352,.F.);
#31631=ORIENTED_EDGE('',*,*,#22193,.T.);
#31632=ORIENTED_EDGE('',*,*,#22153,.F.);
#31633=ORIENTED_EDGE('',*,*,#22156,.F.);
#31634=ORIENTED_EDGE('',*,*,#22350,.F.);
#31635=ORIENTED_EDGE('',*,*,#22150,.F.);
#31636=ORIENTED_EDGE('',*,*,#22353,.T.);
#31637=ORIENTED_EDGE('',*,*,#22354,.T.);
#31638=ORIENTED_EDGE('',*,*,#22355,.T.);
#31639=ORIENTED_EDGE('',*,*,#22353,.F.);
#31640=ORIENTED_EDGE('',*,*,#22356,.T.);
#31641=ORIENTED_EDGE('',*,*,#22116,.T.);
#31642=ORIENTED_EDGE('',*,*,#22357,.T.);
#31643=ORIENTED_EDGE('',*,*,#22356,.F.);
#31644=ORIENTED_EDGE('',*,*,#22358,.F.);
#31645=ORIENTED_EDGE('',*,*,#22359,.F.);
#31646=ORIENTED_EDGE('',*,*,#22351,.T.);
#31647=ORIENTED_EDGE('',*,*,#22117,.F.);
#31648=ORIENTED_EDGE('',*,*,#22355,.F.);
#31649=ORIENTED_EDGE('',*,*,#22360,.T.);
#31650=ORIENTED_EDGE('',*,*,#22361,.F.);
#31651=ORIENTED_EDGE('',*,*,#22358,.T.);
#31652=ORIENTED_EDGE('',*,*,#22354,.F.);
#31653=ORIENTED_EDGE('',*,*,#22362,.T.);
#31654=ORIENTED_EDGE('',*,*,#22363,.F.);
#31655=ORIENTED_EDGE('',*,*,#22364,.T.);
#31656=ORIENTED_EDGE('',*,*,#22365,.T.);
#31657=ORIENTED_EDGE('',*,*,#22366,.T.);
#31658=ORIENTED_EDGE('',*,*,#22367,.T.);
#31659=ORIENTED_EDGE('',*,*,#22196,.T.);
#31660=ORIENTED_EDGE('',*,*,#22368,.T.);
#31661=ORIENTED_EDGE('',*,*,#22369,.T.);
#31662=ORIENTED_EDGE('',*,*,#22370,.T.);
#31663=ORIENTED_EDGE('',*,*,#22195,.T.);
#31664=ORIENTED_EDGE('',*,*,#22370,.F.);
#31665=ORIENTED_EDGE('',*,*,#22363,.T.);
#31666=ORIENTED_EDGE('',*,*,#22365,.F.);
#31667=ORIENTED_EDGE('',*,*,#22371,.T.);
#31668=ORIENTED_EDGE('',*,*,#22194,.T.);
#31669=ORIENTED_EDGE('',*,*,#22352,.T.);
#31670=ORIENTED_EDGE('',*,*,#22359,.T.);
#31671=ORIENTED_EDGE('',*,*,#22371,.F.);
#31672=ORIENTED_EDGE('',*,*,#22361,.T.);
#31673=ORIENTED_EDGE('',*,*,#22368,.F.);
#31674=ORIENTED_EDGE('',*,*,#22369,.F.);
#31675=ORIENTED_EDGE('',*,*,#22360,.F.);
#31676=ORIENTED_EDGE('',*,*,#22364,.F.);
#31677=ORIENTED_EDGE('',*,*,#22357,.F.);
#31678=ORIENTED_EDGE('',*,*,#22115,.F.);
#31679=ORIENTED_EDGE('',*,*,#22372,.F.);
#31680=ORIENTED_EDGE('',*,*,#22366,.F.);
#31681=ORIENTED_EDGE('',*,*,#22362,.F.);
#31682=ORIENTED_EDGE('',*,*,#22373,.T.);
#31683=ORIENTED_EDGE('',*,*,#22374,.T.);
#31684=ORIENTED_EDGE('',*,*,#22375,.T.);
#31685=ORIENTED_EDGE('',*,*,#22373,.F.);
#31686=ORIENTED_EDGE('',*,*,#22376,.T.);
#31687=ORIENTED_EDGE('',*,*,#22107,.T.);
#31688=ORIENTED_EDGE('',*,*,#22377,.T.);
#31689=ORIENTED_EDGE('',*,*,#22376,.F.);
#31690=ORIENTED_EDGE('',*,*,#22378,.F.);
#31691=ORIENTED_EDGE('',*,*,#22205,.T.);
#31692=ORIENTED_EDGE('',*,*,#22379,.T.);
#31693=ORIENTED_EDGE('',*,*,#22108,.F.);
#31694=ORIENTED_EDGE('',*,*,#22375,.F.);
#31695=ORIENTED_EDGE('',*,*,#22380,.T.);
#31696=ORIENTED_EDGE('',*,*,#22381,.T.);
#31697=ORIENTED_EDGE('',*,*,#22206,.T.);
#31698=ORIENTED_EDGE('',*,*,#22378,.T.);
#31699=ORIENTED_EDGE('',*,*,#22374,.F.);
#31700=ORIENTED_EDGE('',*,*,#22382,.T.);
#31701=ORIENTED_EDGE('',*,*,#22208,.T.);
#31702=ORIENTED_EDGE('',*,*,#22383,.T.);
#31703=ORIENTED_EDGE('',*,*,#22384,.T.);
#31704=ORIENTED_EDGE('',*,*,#22385,.T.);
#31705=ORIENTED_EDGE('',*,*,#22386,.T.);
#31706=ORIENTED_EDGE('',*,*,#22387,.T.);
#31707=ORIENTED_EDGE('',*,*,#22385,.F.);
#31708=ORIENTED_EDGE('',*,*,#22388,.T.);
#31709=ORIENTED_EDGE('',*,*,#22110,.T.);
#31710=ORIENTED_EDGE('',*,*,#22389,.T.);
#31711=ORIENTED_EDGE('',*,*,#22388,.F.);
#31712=ORIENTED_EDGE('',*,*,#22390,.F.);
#31713=ORIENTED_EDGE('',*,*,#22200,.T.);
#31714=ORIENTED_EDGE('',*,*,#22391,.F.);
#31715=ORIENTED_EDGE('',*,*,#22392,.T.);
#31716=ORIENTED_EDGE('',*,*,#22111,.F.);
#31717=ORIENTED_EDGE('',*,*,#22387,.F.);
#31718=ORIENTED_EDGE('',*,*,#22393,.T.);
#31719=ORIENTED_EDGE('',*,*,#22394,.T.);
#31720=ORIENTED_EDGE('',*,*,#22201,.T.);
#31721=ORIENTED_EDGE('',*,*,#22390,.T.);
#31722=ORIENTED_EDGE('',*,*,#22386,.F.);
#31723=ORIENTED_EDGE('',*,*,#22395,.T.);
#31724=ORIENTED_EDGE('',*,*,#22203,.T.);
#31725=ORIENTED_EDGE('',*,*,#22396,.T.);
#31726=ORIENTED_EDGE('',*,*,#22397,.T.);
#31727=ORIENTED_EDGE('',*,*,#22398,.T.);
#31728=ORIENTED_EDGE('',*,*,#22399,.T.);
#31729=ORIENTED_EDGE('',*,*,#22400,.T.);
#31730=ORIENTED_EDGE('',*,*,#22398,.F.);
#31731=ORIENTED_EDGE('',*,*,#22401,.T.);
#31732=ORIENTED_EDGE('',*,*,#22113,.T.);
#31733=ORIENTED_EDGE('',*,*,#22402,.T.);
#31734=ORIENTED_EDGE('',*,*,#22401,.F.);
#31735=ORIENTED_EDGE('',*,*,#22403,.F.);
#31736=ORIENTED_EDGE('',*,*,#22404,.F.);
#31737=ORIENTED_EDGE('',*,*,#22372,.T.);
#31738=ORIENTED_EDGE('',*,*,#22114,.F.);
#31739=ORIENTED_EDGE('',*,*,#22400,.F.);
#31740=ORIENTED_EDGE('',*,*,#22405,.T.);
#31741=ORIENTED_EDGE('',*,*,#22406,.F.);
#31742=ORIENTED_EDGE('',*,*,#22403,.T.);
#31743=ORIENTED_EDGE('',*,*,#22399,.F.);
#31744=ORIENTED_EDGE('',*,*,#22407,.T.);
#31745=ORIENTED_EDGE('',*,*,#22408,.F.);
#31746=ORIENTED_EDGE('',*,*,#22409,.T.);
#31747=ORIENTED_EDGE('',*,*,#22410,.T.);
#31748=ORIENTED_EDGE('',*,*,#22411,.T.);
#31749=ORIENTED_EDGE('',*,*,#22391,.T.);
#31750=ORIENTED_EDGE('',*,*,#22199,.T.);
#31751=ORIENTED_EDGE('',*,*,#22412,.T.);
#31752=ORIENTED_EDGE('',*,*,#22413,.T.);
#31753=ORIENTED_EDGE('',*,*,#22414,.T.);
#31754=ORIENTED_EDGE('',*,*,#22198,.T.);
#31755=ORIENTED_EDGE('',*,*,#22414,.F.);
#31756=ORIENTED_EDGE('',*,*,#22408,.T.);
#31757=ORIENTED_EDGE('',*,*,#22410,.F.);
#31758=ORIENTED_EDGE('',*,*,#22415,.T.);
#31759=ORIENTED_EDGE('',*,*,#22197,.T.);
#31760=ORIENTED_EDGE('',*,*,#22367,.F.);
#31761=ORIENTED_EDGE('',*,*,#22404,.T.);
#31762=ORIENTED_EDGE('',*,*,#22415,.F.);
#31763=ORIENTED_EDGE('',*,*,#22406,.T.);
#31764=ORIENTED_EDGE('',*,*,#22412,.F.);
#31765=ORIENTED_EDGE('',*,*,#22413,.F.);
#31766=ORIENTED_EDGE('',*,*,#22405,.F.);
#31767=ORIENTED_EDGE('',*,*,#22409,.F.);
#31768=ORIENTED_EDGE('',*,*,#22402,.F.);
#31769=ORIENTED_EDGE('',*,*,#22112,.F.);
#31770=ORIENTED_EDGE('',*,*,#22392,.F.);
#31771=ORIENTED_EDGE('',*,*,#22411,.F.);
#31772=ORIENTED_EDGE('',*,*,#22407,.F.);
#31773=ORIENTED_EDGE('',*,*,#22202,.T.);
#31774=ORIENTED_EDGE('',*,*,#22394,.F.);
#31775=ORIENTED_EDGE('',*,*,#22416,.T.);
#31776=ORIENTED_EDGE('',*,*,#22396,.F.);
#31777=ORIENTED_EDGE('',*,*,#22389,.F.);
#31778=ORIENTED_EDGE('',*,*,#22109,.F.);
#31779=ORIENTED_EDGE('',*,*,#22379,.F.);
#31780=ORIENTED_EDGE('',*,*,#22204,.T.);
#31781=ORIENTED_EDGE('',*,*,#22395,.F.);
#31782=ORIENTED_EDGE('',*,*,#22397,.F.);
#31783=ORIENTED_EDGE('',*,*,#22416,.F.);
#31784=ORIENTED_EDGE('',*,*,#22393,.F.);
#31785=ORIENTED_EDGE('',*,*,#22207,.T.);
#31786=ORIENTED_EDGE('',*,*,#22381,.F.);
#31787=ORIENTED_EDGE('',*,*,#22417,.T.);
#31788=ORIENTED_EDGE('',*,*,#22383,.F.);
#31789=ORIENTED_EDGE('',*,*,#22377,.F.);
#31790=ORIENTED_EDGE('',*,*,#22106,.F.);
#31791=ORIENTED_EDGE('',*,*,#22298,.F.);
#31792=ORIENTED_EDGE('',*,*,#22250,.F.);
#31793=ORIENTED_EDGE('',*,*,#22209,.T.);
#31794=ORIENTED_EDGE('',*,*,#22382,.F.);
#31795=ORIENTED_EDGE('',*,*,#22384,.F.);
#31796=ORIENTED_EDGE('',*,*,#22417,.F.);
#31797=ORIENTED_EDGE('',*,*,#22380,.F.);
#31798=ORIENTED_EDGE('',*,*,#22174,.F.);
#31799=ORIENTED_EDGE('',*,*,#22121,.F.);
#31800=ORIENTED_EDGE('',*,*,#22149,.F.);
#31801=ORIENTED_EDGE('',*,*,#22180,.F.);
#31802=ORIENTED_EDGE('',*,*,#22176,.F.);
#31803=ORIENTED_EDGE('',*,*,#22306,.F.);
#31804=ORIENTED_EDGE('',*,*,#22347,.T.);
#31805=ORIENTED_EDGE('',*,*,#22135,.F.);
#31806=ORIENTED_EDGE('',*,*,#22315,.F.);
#31807=ORIENTED_EDGE('',*,*,#22321,.F.);
#31808=ORIENTED_EDGE('',*,*,#22322,.F.);
#31809=ORIENTED_EDGE('',*,*,#22346,.T.);
#31810=ORIENTED_EDGE('',*,*,#22132,.F.);
#31811=ORIENTED_EDGE('',*,*,#22331,.F.);
#31812=ORIENTED_EDGE('',*,*,#22337,.F.);
#37666=CYLINDRICAL_SURFACE('',#43005,18.);
#37667=CYLINDRICAL_SURFACE('',#43031,0.4);
#37668=CYLINDRICAL_SURFACE('',#43043,11.05);
#37669=CYLINDRICAL_SURFACE('',#43053,0.4);
#37670=CYLINDRICAL_SURFACE('',#43057,0.4);
#37671=CYLINDRICAL_SURFACE('',#43088,0.4);
#37672=CYLINDRICAL_SURFACE('',#43098,0.4);
#37673=CYLINDRICAL_SURFACE('',#43100,0.4);
#37674=CYLINDRICAL_SURFACE('',#43107,0.4);
#37675=CYLINDRICAL_SURFACE('',#43117,0.4);
#37676=CYLINDRICAL_SURFACE('',#43119,0.4);
#37677=CYLINDRICAL_SURFACE('',#43129,0.4);
#37678=CYLINDRICAL_SURFACE('',#43132,0.4);
#37679=CYLINDRICAL_SURFACE('',#43135,0.4);
#37680=CYLINDRICAL_SURFACE('',#43138,0.4);
#37681=CYLINDRICAL_SURFACE('',#43153,0.4);
#37682=CYLINDRICAL_SURFACE('',#43155,0.4);
#37683=CYLINDRICAL_SURFACE('',#43158,0.4);
#37684=CYLINDRICAL_SURFACE('',#43164,0.4);
#37685=CYLINDRICAL_SURFACE('',#43167,0.4);
#37686=CYLINDRICAL_SURFACE('',#43170,0.4);
#37687=CYLINDRICAL_SURFACE('',#43176,0.4);
#37688=CYLINDRICAL_SURFACE('',#43179,0.4);
#37689=CYLINDRICAL_SURFACE('',#43200,0.4);
#37690=CYLINDRICAL_SURFACE('',#43214,0.4);
#37691=CYLINDRICAL_SURFACE('',#43218,0.4);
#37692=CYLINDRICAL_SURFACE('',#43226,0.4);
#37693=CYLINDRICAL_SURFACE('',#43235,0.4);
#37694=CYLINDRICAL_SURFACE('',#43241,0.4);
#37695=CYLINDRICAL_SURFACE('',#43248,0.4);
#37696=CYLINDRICAL_SURFACE('',#43252,0.4);
#37697=CYLINDRICAL_SURFACE('',#43259,0.4);
#39209=ADVANCED_FACE('',(#3406),#955,.T.);
#39210=ADVANCED_FACE('',(#3407),#37666,.T.);
#39211=ADVANCED_FACE('',(#3408),#673,.T.);
#39212=ADVANCED_FACE('',(#3409),#956,.T.);
#39213=ADVANCED_FACE('',(#3410,#1049),#1302,.T.);
#39214=ADVANCED_FACE('',(#3411),#505,.T.);
#39215=ADVANCED_FACE('',(#3412),#37667,.T.);
#39216=ADVANCED_FACE('',(#3413),#1303,.T.);
#39217=ADVANCED_FACE('',(#3414),#2083,.F.);
#39218=ADVANCED_FACE('',(#3415),#2084,.F.);
#39219=ADVANCED_FACE('',(#3416),#957,.T.);
#39220=ADVANCED_FACE('',(#3417,#1050),#1304,.T.);
#39221=ADVANCED_FACE('',(#3418),#958,.T.);
#39222=ADVANCED_FACE('',(#3419),#37668,.F.);
#39223=ADVANCED_FACE('',(#3420),#959,.T.);
#39224=ADVANCED_FACE('',(#3421),#674,.F.);
#39225=ADVANCED_FACE('',(#3422),#37669,.T.);
#39226=ADVANCED_FACE('',(#3423),#2085,.F.);
#39227=ADVANCED_FACE('',(#3424),#37670,.T.);
#39228=ADVANCED_FACE('',(#3425),#506,.T.);
#39229=ADVANCED_FACE('',(#3426),#507,.T.);
#39230=ADVANCED_FACE('',(#3427),#1305,.T.);
#39231=ADVANCED_FACE('',(#3428),#2086,.F.);
#39232=ADVANCED_FACE('',(#3429),#675,.T.);
#39233=ADVANCED_FACE('',(#3430),#960,.T.);
#39234=ADVANCED_FACE('',(#3431,#1051),#1306,.F.);
#39235=ADVANCED_FACE('',(#3432),#508,.T.);
#39236=ADVANCED_FACE('',(#3433),#2087,.F.);
#39237=ADVANCED_FACE('',(#3434),#37671,.T.);
#39238=ADVANCED_FACE('',(#3435),#2088,.F.);
#39239=ADVANCED_FACE('',(#3436),#509,.T.);
#39240=ADVANCED_FACE('',(#3437),#510,.T.);
#39241=ADVANCED_FACE('',(#3438),#1307,.T.);
#39242=ADVANCED_FACE('',(#3439),#37672,.T.);
#39243=ADVANCED_FACE('',(#3440),#1308,.T.);
#39244=ADVANCED_FACE('',(#3441),#37673,.T.);
#39245=ADVANCED_FACE('',(#3442),#2089,.F.);
#39246=ADVANCED_FACE('',(#3443),#511,.T.);
#39247=ADVANCED_FACE('',(#3444),#37674,.T.);
#39248=ADVANCED_FACE('',(#3445),#512,.T.);
#39249=ADVANCED_FACE('',(#3446),#961,.T.);
#39250=ADVANCED_FACE('',(#3447),#676,.T.);
#39251=ADVANCED_FACE('',(#3448),#2090,.F.);
#39252=ADVANCED_FACE('',(#3449),#1309,.T.);
#39253=ADVANCED_FACE('',(#3450),#37675,.T.);
#39254=ADVANCED_FACE('',(#3451),#2091,.F.);
#39255=ADVANCED_FACE('',(#3452),#37676,.T.);
#39256=ADVANCED_FACE('',(#3453),#513,.T.);
#39257=ADVANCED_FACE('',(#3454),#1310,.T.);
#39258=ADVANCED_FACE('',(#3455),#677,.T.);
#39259=ADVANCED_FACE('',(#3456),#962,.T.);
#39260=ADVANCED_FACE('',(#3457),#678,.T.);
#39261=ADVANCED_FACE('',(#3458),#37677,.T.);
#39262=ADVANCED_FACE('',(#3459),#963,.T.);
#39263=ADVANCED_FACE('',(#3460),#37678,.T.);
#39264=ADVANCED_FACE('',(#3461),#1311,.T.);
#39265=ADVANCED_FACE('',(#3462),#37679,.T.);
#39266=ADVANCED_FACE('',(#3463),#37680,.T.);
#39267=ADVANCED_FACE('',(#3464),#2092,.F.);
#39268=ADVANCED_FACE('',(#3465),#514,.T.);
#39269=ADVANCED_FACE('',(#3466),#515,.T.);
#39270=ADVANCED_FACE('',(#3467),#516,.T.);
#39271=ADVANCED_FACE('',(#3468),#1312,.T.);
#39272=ADVANCED_FACE('',(#3469),#964,.T.);
#39273=ADVANCED_FACE('',(#3470),#679,.T.);
#39274=ADVANCED_FACE('',(#3471),#37681,.T.);
#39275=ADVANCED_FACE('',(#3472),#2093,.F.);
#39276=ADVANCED_FACE('',(#3473),#37682,.T.);
#39277=ADVANCED_FACE('',(#3474),#37683,.T.);
#39278=ADVANCED_FACE('',(#3475),#517,.T.);
#39279=ADVANCED_FACE('',(#3476),#37684,.T.);
#39280=ADVANCED_FACE('',(#3477),#2094,.F.);
#39281=ADVANCED_FACE('',(#3478),#2095,.F.);
#39282=ADVANCED_FACE('',(#3479),#37685,.T.);
#39283=ADVANCED_FACE('',(#3480),#37686,.T.);
#39284=ADVANCED_FACE('',(#3481),#518,.T.);
#39285=ADVANCED_FACE('',(#3482),#37687,.T.);
#39286=ADVANCED_FACE('',(#3483),#2096,.F.);
#39287=ADVANCED_FACE('',(#3484),#2097,.F.);
#39288=ADVANCED_FACE('',(#3485),#37688,.T.);
#39289=ADVANCED_FACE('',(#3486),#519,.T.);
#39290=ADVANCED_FACE('',(#3487),#520,.T.);
#39291=ADVANCED_FACE('',(#3488),#521,.T.);
#39292=ADVANCED_FACE('',(#3489),#522,.T.);
#39293=ADVANCED_FACE('',(#3490),#523,.T.);
#39294=ADVANCED_FACE('',(#3491),#1313,.T.);
#39295=ADVANCED_FACE('',(#3492),#680,.T.);
#39296=ADVANCED_FACE('',(#3493),#965,.T.);
#39297=ADVANCED_FACE('',(#3494),#681,.T.);
#39298=ADVANCED_FACE('',(#3495),#966,.T.);
#39299=ADVANCED_FACE('',(#3496),#1314,.T.);
#39300=ADVANCED_FACE('',(#3497),#1315,.T.);
#39301=ADVANCED_FACE('',(#3498),#1316,.T.);
#39302=ADVANCED_FACE('',(#3499),#37689,.T.);
#39303=ADVANCED_FACE('',(#3500),#524,.T.);
#39304=ADVANCED_FACE('',(#3501),#967,.T.);
#39305=ADVANCED_FACE('',(#3502),#968,.T.);
#39306=ADVANCED_FACE('',(#3503),#1317,.T.);
#39307=ADVANCED_FACE('',(#3504),#682,.T.);
#39308=ADVANCED_FACE('',(#3505),#525,.T.);
#39309=ADVANCED_FACE('',(#3506),#37690,.T.);
#39310=ADVANCED_FACE('',(#3507),#1318,.T.);
#39311=ADVANCED_FACE('',(#3508),#2098,.F.);
#39312=ADVANCED_FACE('',(#3509),#2099,.F.);
#39313=ADVANCED_FACE('',(#3510),#37691,.T.);
#39314=ADVANCED_FACE('',(#3511),#969,.T.);
#39315=ADVANCED_FACE('',(#3512),#526,.T.);
#39316=ADVANCED_FACE('',(#3513),#37692,.T.);
#39317=ADVANCED_FACE('',(#3514),#527,.T.);
#39318=ADVANCED_FACE('',(#3515),#683,.T.);
#39319=ADVANCED_FACE('',(#3516),#1319,.T.);
#39320=ADVANCED_FACE('',(#3517),#528,.T.);
#39321=ADVANCED_FACE('',(#3518),#37693,.T.);
#39322=ADVANCED_FACE('',(#3519),#1320,.T.);
#39323=ADVANCED_FACE('',(#3520),#2100,.F.);
#39324=ADVANCED_FACE('',(#3521),#2101,.F.);
#39325=ADVANCED_FACE('',(#3522),#529,.T.);
#39326=ADVANCED_FACE('',(#3523),#37694,.T.);
#39327=ADVANCED_FACE('',(#3524),#1321,.T.);
#39328=ADVANCED_FACE('',(#3525),#2102,.F.);
#39329=ADVANCED_FACE('',(#3526),#2103,.F.);
#39330=ADVANCED_FACE('',(#3527),#530,.T.);
#39331=ADVANCED_FACE('',(#3528),#37695,.T.);
#39332=ADVANCED_FACE('',(#3529),#1322,.T.);
#39333=ADVANCED_FACE('',(#3530),#2104,.F.);
#39334=ADVANCED_FACE('',(#3531),#2105,.F.);
#39335=ADVANCED_FACE('',(#3532),#37696,.T.);
#39336=ADVANCED_FACE('',(#3533),#970,.T.);
#39337=ADVANCED_FACE('',(#3534),#531,.T.);
#39338=ADVANCED_FACE('',(#3535),#37697,.T.);
#39339=ADVANCED_FACE('',(#3536),#532,.T.);
#39340=ADVANCED_FACE('',(#3537),#684,.T.);
#39341=ADVANCED_FACE('',(#3538),#1323,.T.);
#39342=ADVANCED_FACE('',(#3539),#971,.T.);
#39343=ADVANCED_FACE('',(#3540),#1324,.T.);
#39344=ADVANCED_FACE('',(#3541),#685,.T.);
#39345=ADVANCED_FACE('',(#3542),#972,.T.);
#39346=ADVANCED_FACE('',(#3543),#1325,.T.);
#39347=ADVANCED_FACE('',(#3544),#686,.T.);
#39348=ADVANCED_FACE('',(#3545),#1326,.T.);
#39349=ADVANCED_FACE('',(#3546),#1327,.T.);
#39350=ADVANCED_FACE('',(#3547),#1328,.T.);
#40347=CLOSED_SHELL('',(#39209,#39210,#39211,#39212,#39213,#39214,#39215,
#39216,#39217,#39218,#39219,#39220,#39221,#39222,#39223,#39224,#39225,#39226,
#39227,#39228,#39229,#39230,#39231,#39232,#39233,#39234,#39235,#39236,#39237,
#39238,#39239,#39240,#39241,#39242,#39243,#39244,#39245,#39246,#39247,#39248,
#39249,#39250,#39251,#39252,#39253,#39254,#39255,#39256,#39257,#39258,#39259,
#39260,#39261,#39262,#39263,#39264,#39265,#39266,#39267,#39268,#39269,#39270,
#39271,#39272,#39273,#39274,#39275,#39276,#39277,#39278,#39279,#39280,#39281,
#39282,#39283,#39284,#39285,#39286,#39287,#39288,#39289,#39290,#39291,#39292,
#39293,#39294,#39295,#39296,#39297,#39298,#39299,#39300,#39301,#39302,#39303,
#39304,#39305,#39306,#39307,#39308,#39309,#39310,#39311,#39312,#39313,#39314,
#39315,#39316,#39317,#39318,#39319,#39320,#39321,#39322,#39323,#39324,#39325,
#39326,#39327,#39328,#39329,#39330,#39331,#39332,#39333,#39334,#39335,#39336,
#39337,#39338,#39339,#39340,#39341,#39342,#39343,#39344,#39345,#39346,#39347,
#39348,#39349,#39350));
#42998=AXIS2_PLACEMENT_3D('',#77126,#51227,#51228);
#42999=AXIS2_PLACEMENT_3D('',#77127,#51229,#51230);
#43000=AXIS2_PLACEMENT_3D('',#77130,#51231,#51232);
#43001=AXIS2_PLACEMENT_3D('',#77131,#51233,#51234);
#43002=AXIS2_PLACEMENT_3D('',#77133,#51235,#51236);
#43003=AXIS2_PLACEMENT_3D('',#77135,#51237,#51238);
#43004=AXIS2_PLACEMENT_3D('',#77136,#51239,#51240);
#43005=AXIS2_PLACEMENT_3D('',#77137,#51241,#51242);
#43006=AXIS2_PLACEMENT_3D('',#77141,#51244,#51245);
#43007=AXIS2_PLACEMENT_3D('',#77142,#51246,#51247);
#43008=AXIS2_PLACEMENT_3D('',#77143,#51248,#51249);
#43009=AXIS2_PLACEMENT_3D('',#77146,#51250,#51251);
#43010=AXIS2_PLACEMENT_3D('',#77148,#51253,#51254);
#43011=AXIS2_PLACEMENT_3D('',#77149,#51255,#51256);
#43012=AXIS2_PLACEMENT_3D('',#77151,#51257,#51258);
#43013=AXIS2_PLACEMENT_3D('',#77152,#51259,#51260);
#43014=AXIS2_PLACEMENT_3D('',#77153,#51261,#51262);
#43015=AXIS2_PLACEMENT_3D('',#77160,#51265,#51266);
#43016=AXIS2_PLACEMENT_3D('',#77166,#51269,#51270);
#43017=AXIS2_PLACEMENT_3D('',#77172,#51273,#51274);
#43018=AXIS2_PLACEMENT_3D('',#77178,#51277,#51278);
#43019=AXIS2_PLACEMENT_3D('',#77184,#51281,#51282);
#43020=AXIS2_PLACEMENT_3D('',#77190,#51285,#51286);
#43021=AXIS2_PLACEMENT_3D('',#77196,#51289,#51290);
#43022=AXIS2_PLACEMENT_3D('',#77202,#51293,#51294);
#43023=AXIS2_PLACEMENT_3D('',#77208,#51297,#51298);
#43024=AXIS2_PLACEMENT_3D('',#77214,#51301,#51302);
#43025=AXIS2_PLACEMENT_3D('',#77220,#51305,#51306);
#43026=AXIS2_PLACEMENT_3D('',#77225,#51309,#51310);
#43027=AXIS2_PLACEMENT_3D('',#77226,#51311,#51312);
#43028=AXIS2_PLACEMENT_3D('',#77229,#51313,#51314);
#43029=AXIS2_PLACEMENT_3D('',#77231,#51315,#51316);
#43030=AXIS2_PLACEMENT_3D('',#77232,#51317,#51318);
#43031=AXIS2_PLACEMENT_3D('',#77233,#51319,#51320);
#43032=AXIS2_PLACEMENT_3D('',#77236,#51323,#51324);
#43033=AXIS2_PLACEMENT_3D('',#77245,#51326,#51327);
#43034=AXIS2_PLACEMENT_3D('',#77322,#51329,#51330);
#43035=AXIS2_PLACEMENT_3D('',#77324,#51331,#51332);
#43036=AXIS2_PLACEMENT_3D('',#77325,#51333,#51334);
#43037=AXIS2_PLACEMENT_3D('',#77326,#51335,#51336);
#43038=AXIS2_PLACEMENT_3D('',#77328,#51337,#51338);
#43039=AXIS2_PLACEMENT_3D('',#77329,#51339,#51340);
#43040=AXIS2_PLACEMENT_3D('',#77332,#51341,#51342);
#43041=AXIS2_PLACEMENT_3D('',#77333,#51343,#51344);
#43042=AXIS2_PLACEMENT_3D('',#77334,#51345,#51346);
#43043=AXIS2_PLACEMENT_3D('',#77335,#51347,#51348);
#43044=AXIS2_PLACEMENT_3D('',#77339,#51350,#51351);
#43045=AXIS2_PLACEMENT_3D('',#77340,#51352,#51353);
#43046=AXIS2_PLACEMENT_3D('',#77341,#51354,#51355);
#43047=AXIS2_PLACEMENT_3D('',#77344,#51356,#51357);
#43048=AXIS2_PLACEMENT_3D('',#77345,#51358,#51359);
#43049=AXIS2_PLACEMENT_3D('',#77346,#51360,#51361);
#43050=AXIS2_PLACEMENT_3D('',#77347,#51362,#51363);
#43051=AXIS2_PLACEMENT_3D('',#77350,#51364,#51365);
#43052=AXIS2_PLACEMENT_3D('',#77352,#51367,#51368);
#43053=AXIS2_PLACEMENT_3D('',#77353,#51369,#51370);
#43054=AXIS2_PLACEMENT_3D('',#77356,#51371,#51372);
#43055=AXIS2_PLACEMENT_3D('',#77376,#51375,#51376);
#43056=AXIS2_PLACEMENT_3D('',#77383,#51377,#51378);
#43057=AXIS2_PLACEMENT_3D('',#77388,#51379,#51380);
#43058=AXIS2_PLACEMENT_3D('',#77390,#51381,#51382);
#43059=AXIS2_PLACEMENT_3D('',#77393,#51385,#51386);
#43060=AXIS2_PLACEMENT_3D('',#77394,#51387,#51388);
#43061=AXIS2_PLACEMENT_3D('',#77395,#51389,#51390);
#43062=AXIS2_PLACEMENT_3D('',#77396,#51391,#51392);
#43063=AXIS2_PLACEMENT_3D('',#77397,#51393,#51394);
#43064=AXIS2_PLACEMENT_3D('',#77427,#51397,#51398);
#43065=AXIS2_PLACEMENT_3D('',#77428,#51399,#51400);
#43066=AXIS2_PLACEMENT_3D('',#77429,#51401,#51402);
#43067=AXIS2_PLACEMENT_3D('',#77430,#51403,#51404);
#43068=AXIS2_PLACEMENT_3D('',#77432,#51405,#51406);
#43069=AXIS2_PLACEMENT_3D('',#77433,#51407,#51408);
#43070=AXIS2_PLACEMENT_3D('',#77434,#51409,#51410);
#43071=AXIS2_PLACEMENT_3D('',#77435,#51411,#51412);
#43072=AXIS2_PLACEMENT_3D('',#77441,#51415,#51416);
#43073=AXIS2_PLACEMENT_3D('',#77447,#51419,#51420);
#43074=AXIS2_PLACEMENT_3D('',#77461,#51423,#51424);
#43075=AXIS2_PLACEMENT_3D('',#77483,#51427,#51428);
#43076=AXIS2_PLACEMENT_3D('',#77497,#51431,#51432);
#43077=AXIS2_PLACEMENT_3D('',#77503,#51435,#51436);
#43078=AXIS2_PLACEMENT_3D('',#77509,#51439,#51440);
#43079=AXIS2_PLACEMENT_3D('',#77515,#51443,#51444);
#43080=AXIS2_PLACEMENT_3D('',#77521,#51447,#51448);
#43081=AXIS2_PLACEMENT_3D('',#77527,#51451,#51452);
#43082=AXIS2_PLACEMENT_3D('',#77532,#51455,#51456);
#43083=AXIS2_PLACEMENT_3D('',#77533,#51457,#51458);
#43084=AXIS2_PLACEMENT_3D('',#77536,#51459,#51460);
#43085=AXIS2_PLACEMENT_3D('',#77537,#51461,#51462);
#43086=AXIS2_PLACEMENT_3D('',#77538,#51463,#51464);
#43087=AXIS2_PLACEMENT_3D('',#77557,#51465,#51466);
#43088=AXIS2_PLACEMENT_3D('',#77566,#51467,#51468);
#43089=AXIS2_PLACEMENT_3D('',#77568,#51469,#51470);
#43090=AXIS2_PLACEMENT_3D('',#77570,#51471,#51472);
#43091=AXIS2_PLACEMENT_3D('',#77589,#51474,#51475);
#43092=AXIS2_PLACEMENT_3D('',#77595,#51476,#51477);
#43093=AXIS2_PLACEMENT_3D('',#77600,#51478,#51479);
#43094=AXIS2_PLACEMENT_3D('',#77601,#51480,#51481);
#43095=AXIS2_PLACEMENT_3D('',#77602,#51482,#51483);
#43096=AXIS2_PLACEMENT_3D('',#77603,#51484,#51485);
#43097=AXIS2_PLACEMENT_3D('',#77604,#51486,#51487);
#43098=AXIS2_PLACEMENT_3D('',#77607,#51490,#51491);
#43099=AXIS2_PLACEMENT_3D('',#77609,#51493,#51494);
#43100=AXIS2_PLACEMENT_3D('',#77611,#51496,#51497);
#43101=AXIS2_PLACEMENT_3D('',#77613,#51498,#51499);
#43102=AXIS2_PLACEMENT_3D('',#77615,#51500,#51501);
#43103=AXIS2_PLACEMENT_3D('',#77634,#51503,#51504);
#43104=AXIS2_PLACEMENT_3D('',#77641,#51505,#51506);
#43105=AXIS2_PLACEMENT_3D('',#77646,#51507,#51508);
#43106=AXIS2_PLACEMENT_3D('',#77647,#51509,#51510);
#43107=AXIS2_PLACEMENT_3D('',#77648,#51511,#51512);
#43108=AXIS2_PLACEMENT_3D('',#77650,#51513,#51514);
#43109=AXIS2_PLACEMENT_3D('',#77653,#51517,#51518);
#43110=AXIS2_PLACEMENT_3D('',#77654,#51519,#51520);
#43111=AXIS2_PLACEMENT_3D('',#77655,#51521,#51522);
#43112=AXIS2_PLACEMENT_3D('',#77657,#51523,#51524);
#43113=AXIS2_PLACEMENT_3D('',#77658,#51525,#51526);
#43114=AXIS2_PLACEMENT_3D('',#77659,#51527,#51528);
#43115=AXIS2_PLACEMENT_3D('',#77685,#51529,#51530);
#43116=AXIS2_PLACEMENT_3D('',#77686,#51531,#51532);
#43117=AXIS2_PLACEMENT_3D('',#77690,#51535,#51536);
#43118=AXIS2_PLACEMENT_3D('',#77747,#51539,#51540);
#43119=AXIS2_PLACEMENT_3D('',#77752,#51541,#51542);
#43120=AXIS2_PLACEMENT_3D('',#77753,#51543,#51544);
#43121=AXIS2_PLACEMENT_3D('',#77755,#51546,#51547);
#43122=AXIS2_PLACEMENT_3D('',#77756,#51548,#51549);
#43123=AXIS2_PLACEMENT_3D('',#77757,#51550,#51551);
#43124=AXIS2_PLACEMENT_3D('',#77765,#51554,#51555);
#43125=AXIS2_PLACEMENT_3D('',#77767,#51556,#51557);
#43126=AXIS2_PLACEMENT_3D('',#77783,#51558,#51559);
#43127=AXIS2_PLACEMENT_3D('',#77792,#51560,#51561);
#43128=AXIS2_PLACEMENT_3D('',#77793,#51562,#51563);
#43129=AXIS2_PLACEMENT_3D('',#77794,#51564,#51565);
#43130=AXIS2_PLACEMENT_3D('',#77795,#51566,#51567);
#43131=AXIS2_PLACEMENT_3D('',#77796,#51568,#51569);
#43132=AXIS2_PLACEMENT_3D('',#77797,#51570,#51571);
#43133=AXIS2_PLACEMENT_3D('',#77798,#51572,#51573);
#43134=AXIS2_PLACEMENT_3D('',#77799,#51574,#51575);
#43135=AXIS2_PLACEMENT_3D('',#77800,#51576,#51577);
#43136=AXIS2_PLACEMENT_3D('',#77803,#51579,#51580);
#43137=AXIS2_PLACEMENT_3D('',#77804,#51581,#51582);
#43138=AXIS2_PLACEMENT_3D('',#77805,#51583,#51584);
#43139=AXIS2_PLACEMENT_3D('',#77806,#51585,#51586);
#43140=AXIS2_PLACEMENT_3D('',#77824,#51587,#51588);
#43141=AXIS2_PLACEMENT_3D('',#77831,#51589,#51590);
#43142=AXIS2_PLACEMENT_3D('',#77836,#51591,#51592);
#43143=AXIS2_PLACEMENT_3D('',#77838,#51593,#51594);
#43144=AXIS2_PLACEMENT_3D('',#77839,#51595,#51596);
#43145=AXIS2_PLACEMENT_3D('',#77840,#51597,#51598);
#43146=AXIS2_PLACEMENT_3D('',#77841,#51599,#51600);
#43147=AXIS2_PLACEMENT_3D('',#77842,#51601,#51602);
#43148=AXIS2_PLACEMENT_3D('',#77843,#51603,#51604);
#43149=AXIS2_PLACEMENT_3D('',#77845,#51606,#51607);
#43150=AXIS2_PLACEMENT_3D('',#77847,#51608,#51609);
#43151=AXIS2_PLACEMENT_3D('',#77848,#51610,#51611);
#43152=AXIS2_PLACEMENT_3D('',#77849,#51612,#51613);
#43153=AXIS2_PLACEMENT_3D('',#77854,#51614,#51615);
#43154=AXIS2_PLACEMENT_3D('',#77878,#51618,#51619);
#43155=AXIS2_PLACEMENT_3D('',#77879,#51620,#51621);
#43156=AXIS2_PLACEMENT_3D('',#77883,#51623,#51624);
#43157=AXIS2_PLACEMENT_3D('',#77884,#51625,#51626);
#43158=AXIS2_PLACEMENT_3D('',#77885,#51627,#51628);
#43159=AXIS2_PLACEMENT_3D('',#77886,#51629,#51630);
#43160=AXIS2_PLACEMENT_3D('',#77888,#51632,#51633);
#43161=AXIS2_PLACEMENT_3D('',#77891,#51634,#51635);
#43162=AXIS2_PLACEMENT_3D('',#77893,#51636,#51637);
#43163=AXIS2_PLACEMENT_3D('',#77894,#51638,#51639);
#43164=AXIS2_PLACEMENT_3D('',#77895,#51640,#51641);
#43165=AXIS2_PLACEMENT_3D('',#77920,#51644,#51645);
#43166=AXIS2_PLACEMENT_3D('',#77946,#51646,#51647);
#43167=AXIS2_PLACEMENT_3D('',#77951,#51648,#51649);
#43168=AXIS2_PLACEMENT_3D('',#77955,#51651,#51652);
#43169=AXIS2_PLACEMENT_3D('',#77956,#51653,#51654);
#43170=AXIS2_PLACEMENT_3D('',#77957,#51655,#51656);
#43171=AXIS2_PLACEMENT_3D('',#77958,#51657,#51658);
#43172=AXIS2_PLACEMENT_3D('',#77960,#51660,#51661);
#43173=AXIS2_PLACEMENT_3D('',#77963,#51662,#51663);
#43174=AXIS2_PLACEMENT_3D('',#77965,#51664,#51665);
#43175=AXIS2_PLACEMENT_3D('',#77966,#51666,#51667);
#43176=AXIS2_PLACEMENT_3D('',#77967,#51668,#51669);
#43177=AXIS2_PLACEMENT_3D('',#77992,#51672,#51673);
#43178=AXIS2_PLACEMENT_3D('',#78018,#51674,#51675);
#43179=AXIS2_PLACEMENT_3D('',#78023,#51676,#51677);
#43180=AXIS2_PLACEMENT_3D('',#78024,#51678,#51679);
#43181=AXIS2_PLACEMENT_3D('',#78026,#51681,#51682);
#43182=AXIS2_PLACEMENT_3D('',#78027,#51683,#51684);
#43183=AXIS2_PLACEMENT_3D('',#78028,#51685,#51686);
#43184=AXIS2_PLACEMENT_3D('',#78029,#51687,#51688);
#43185=AXIS2_PLACEMENT_3D('',#78030,#51689,#51690);
#43186=AXIS2_PLACEMENT_3D('',#78031,#51691,#51692);
#43187=AXIS2_PLACEMENT_3D('',#78032,#51693,#51694);
#43188=AXIS2_PLACEMENT_3D('',#78033,#51695,#51696);
#43189=AXIS2_PLACEMENT_3D('',#78034,#51697,#51698);
#43190=AXIS2_PLACEMENT_3D('',#78035,#51699,#51700);
#43191=AXIS2_PLACEMENT_3D('',#78036,#51701,#51702);
#43192=AXIS2_PLACEMENT_3D('',#78037,#51703,#51704);
#43193=AXIS2_PLACEMENT_3D('',#78038,#51705,#51706);
#43194=AXIS2_PLACEMENT_3D('',#78039,#51707,#51708);
#43195=AXIS2_PLACEMENT_3D('',#78040,#51709,#51710);
#43196=AXIS2_PLACEMENT_3D('',#78041,#51711,#51712);
#43197=AXIS2_PLACEMENT_3D('',#78042,#51713,#51714);
#43198=AXIS2_PLACEMENT_3D('',#78043,#51715,#51716);
#43199=AXIS2_PLACEMENT_3D('',#78045,#51718,#51719);
#43200=AXIS2_PLACEMENT_3D('',#78047,#51721,#51722);
#43201=AXIS2_PLACEMENT_3D('',#78048,#51723,#51724);
#43202=AXIS2_PLACEMENT_3D('',#78049,#51725,#51726);
#43203=AXIS2_PLACEMENT_3D('',#78050,#51727,#51728);
#43204=AXIS2_PLACEMENT_3D('',#78051,#51729,#51730);
#43205=AXIS2_PLACEMENT_3D('',#78052,#51731,#51732);
#43206=AXIS2_PLACEMENT_3D('',#78053,#51733,#51734);
#43207=AXIS2_PLACEMENT_3D('',#78054,#51735,#51736);
#43208=AXIS2_PLACEMENT_3D('',#78057,#51738,#51739);
#43209=AXIS2_PLACEMENT_3D('',#78058,#51740,#51741);
#43210=AXIS2_PLACEMENT_3D('',#78059,#51742,#51743);
#43211=AXIS2_PLACEMENT_3D('',#78062,#51744,#51745);
#43212=AXIS2_PLACEMENT_3D('',#78064,#51746,#51747);
#43213=AXIS2_PLACEMENT_3D('',#78065,#51748,#51749);
#43214=AXIS2_PLACEMENT_3D('',#78066,#51750,#51751);
#43215=AXIS2_PLACEMENT_3D('',#78069,#51754,#51755);
#43216=AXIS2_PLACEMENT_3D('',#78097,#51757,#51758);
#43217=AXIS2_PLACEMENT_3D('',#78120,#51759,#51760);
#43218=AXIS2_PLACEMENT_3D('',#78125,#51761,#51762);
#43219=AXIS2_PLACEMENT_3D('',#78126,#51763,#51764);
#43220=AXIS2_PLACEMENT_3D('',#78129,#51766,#51767);
#43221=AXIS2_PLACEMENT_3D('',#78130,#51768,#51769);
#43222=AXIS2_PLACEMENT_3D('',#78131,#51770,#51771);
#43223=AXIS2_PLACEMENT_3D('',#78132,#51772,#51773);
#43224=AXIS2_PLACEMENT_3D('',#78133,#51774,#51775);
#43225=AXIS2_PLACEMENT_3D('',#78134,#51776,#51777);
#43226=AXIS2_PLACEMENT_3D('',#78135,#51778,#51779);
#43227=AXIS2_PLACEMENT_3D('',#78136,#51780,#51781);
#43228=AXIS2_PLACEMENT_3D('',#78137,#51782,#51783);
#43229=AXIS2_PLACEMENT_3D('',#78138,#51784,#51785);
#43230=AXIS2_PLACEMENT_3D('',#78139,#51786,#51787);
#43231=AXIS2_PLACEMENT_3D('',#78141,#51789,#51790);
#43232=AXIS2_PLACEMENT_3D('',#78144,#51791,#51792);
#43233=AXIS2_PLACEMENT_3D('',#78146,#51793,#51794);
#43234=AXIS2_PLACEMENT_3D('',#78147,#51795,#51796);
#43235=AXIS2_PLACEMENT_3D('',#78148,#51797,#51798);
#43236=AXIS2_PLACEMENT_3D('',#78151,#51801,#51802);
#43237=AXIS2_PLACEMENT_3D('',#78215,#51804,#51805);
#43238=AXIS2_PLACEMENT_3D('',#78218,#51806,#51807);
#43239=AXIS2_PLACEMENT_3D('',#78220,#51808,#51809);
#43240=AXIS2_PLACEMENT_3D('',#78221,#51810,#51811);
#43241=AXIS2_PLACEMENT_3D('',#78222,#51812,#51813);
#43242=AXIS2_PLACEMENT_3D('',#78225,#51816,#51817);
#43243=AXIS2_PLACEMENT_3D('',#78231,#51818,#51819);
#43244=AXIS2_PLACEMENT_3D('',#78291,#51821,#51822);
#43245=AXIS2_PLACEMENT_3D('',#78294,#51823,#51824);
#43246=AXIS2_PLACEMENT_3D('',#78296,#51825,#51826);
#43247=AXIS2_PLACEMENT_3D('',#78297,#51827,#51828);
#43248=AXIS2_PLACEMENT_3D('',#78298,#51829,#51830);
#43249=AXIS2_PLACEMENT_3D('',#78301,#51833,#51834);
#43250=AXIS2_PLACEMENT_3D('',#78329,#51836,#51837);
#43251=AXIS2_PLACEMENT_3D('',#78352,#51838,#51839);
#43252=AXIS2_PLACEMENT_3D('',#78357,#51840,#51841);
#43253=AXIS2_PLACEMENT_3D('',#78358,#51842,#51843);
#43254=AXIS2_PLACEMENT_3D('',#78360,#51845,#51846);
#43255=AXIS2_PLACEMENT_3D('',#78361,#51847,#51848);
#43256=AXIS2_PLACEMENT_3D('',#78362,#51849,#51850);
#43257=AXIS2_PLACEMENT_3D('',#78363,#51851,#51852);
#43258=AXIS2_PLACEMENT_3D('',#78364,#51853,#51854);
#43259=AXIS2_PLACEMENT_3D('',#78365,#51855,#51856);
#43260=AXIS2_PLACEMENT_3D('',#78366,#51857,#51858);
#43261=AXIS2_PLACEMENT_3D('',#78367,#51859,#51860);
#43262=AXIS2_PLACEMENT_3D('',#78368,#51861,#51862);
#43263=AXIS2_PLACEMENT_3D('',#78369,#51863,#51864);
#43264=AXIS2_PLACEMENT_3D('',#78370,#51865,#51866);
#43265=AXIS2_PLACEMENT_3D('',#78371,#51867,#51868);
#43266=AXIS2_PLACEMENT_3D('',#78372,#51869,#51870);
#43267=AXIS2_PLACEMENT_3D('',#78373,#51871,#51872);
#43268=AXIS2_PLACEMENT_3D('',#78374,#51873,#51874);
#43269=AXIS2_PLACEMENT_3D('',#78375,#51875,#51876);
#43270=AXIS2_PLACEMENT_3D('',#78376,#51877,#51878);
#43271=AXIS2_PLACEMENT_3D('',#78377,#51879,#51880);
#43272=AXIS2_PLACEMENT_3D('',#78378,#51881,#51882);
#43273=AXIS2_PLACEMENT_3D('',#78379,#51883,#51884);
#43274=AXIS2_PLACEMENT_3D('',#78380,#51885,#51886);
#51227=DIRECTION('axis',(0.,0.,1.));
#51228=DIRECTION('refdir',(1.,0.,0.));
#51229=DIRECTION('center_axis',(1.,0.,0.));
#51230=DIRECTION('ref_axis',(0.,0.,-1.));
#51231=DIRECTION('center_axis',(-1.,0.,0.));
#51232=DIRECTION('ref_axis',(0.,-1.,3.06161699786838E-17));
#51233=DIRECTION('center_axis',(-1.,0.,0.));
#51234=DIRECTION('ref_axis',(0.,-1.,3.06161699786838E-17));
#51235=DIRECTION('center_axis',(0.,-1.,-1.22464679914735E-16));
#51236=DIRECTION('ref_axis',(0.,-1.22464679914735E-16,1.));
#51237=DIRECTION('center_axis',(1.,0.,0.));
#51238=DIRECTION('ref_axis',(0.,-1.,1.83697019872103E-16));
#51239=DIRECTION('center_axis',(1.,0.,0.));
#51240=DIRECTION('ref_axis',(0.,-1.,1.83697019872103E-16));
#51241=DIRECTION('center_axis',(1.,0.,0.));
#51242=DIRECTION('ref_axis',(0.,1.,0.));
#51243=DIRECTION('',(-1.,0.,0.));
#51244=DIRECTION('center_axis',(-1.,0.,0.));
#51245=DIRECTION('ref_axis',(0.,-1.,1.83697019872103E-16));
#51246=DIRECTION('center_axis',(-1.,0.,0.));
#51247=DIRECTION('ref_axis',(0.,-1.,1.83697019872103E-16));
#51248=DIRECTION('center_axis',(-1.,0.,0.));
#51249=DIRECTION('ref_axis',(0.,1.,0.));
#51250=DIRECTION('center_axis',(1.,0.,0.));
#51251=DIRECTION('ref_axis',(0.,-1.,3.06161699786838E-17));
#51252=DIRECTION('',(-0.707106781186547,-0.707106781186548,-8.65956056235493E-17));
#51253=DIRECTION('center_axis',(1.,0.,0.));
#51254=DIRECTION('ref_axis',(0.,-1.,3.06161699786838E-17));
#51255=DIRECTION('center_axis',(1.,0.,0.));
#51256=DIRECTION('ref_axis',(0.,0.,-1.));
#51257=DIRECTION('center_axis',(0.,-1.,-1.22464679914735E-16));
#51258=DIRECTION('ref_axis',(0.,-1.22464679914735E-16,1.));
#51259=DIRECTION('center_axis',(1.,0.,0.));
#51260=DIRECTION('ref_axis',(0.,-1.,1.83697019872103E-16));
#51261=DIRECTION('center_axis',(-1.,0.,0.));
#51262=DIRECTION('ref_axis',(0.,0.,1.));
#51263=DIRECTION('',(0.,-0.00883884484604825,0.999960936647921));
#51264=DIRECTION('',(0.,0.507635132500748,0.861572151506157));
#51265=DIRECTION('center_axis',(1.,0.,0.));
#51266=DIRECTION('ref_axis',(0.,1.,-2.51679948241167E-16));
#51267=DIRECTION('',(0.,-0.507635132500748,0.861572151506157));
#51268=DIRECTION('',(0.,0.00883884484604973,0.999960936647921));
#51269=DIRECTION('center_axis',(1.,0.,0.));
#51270=DIRECTION('ref_axis',(0.,0.866025403784438,0.500000000000001));
#51271=DIRECTION('',(0.,-0.870410996352206,0.492325804147173));
#51272=DIRECTION('',(0.,-0.492325804147172,0.870410996352206));
#51273=DIRECTION('center_axis',(1.,0.,0.));
#51274=DIRECTION('ref_axis',(0.,0.500000000000001,0.866025403784438));
#51275=DIRECTION('',(0.,-0.999960936647921,-0.00883884484604923));
#51276=DIRECTION('',(0.,-0.861572151506157,0.507635132500748));
#51277=DIRECTION('center_axis',(1.,0.,0.));
#51278=DIRECTION('ref_axis',(0.,2.51679948241167E-16,1.));
#51279=DIRECTION('',(0.,-0.861572151506157,-0.507635132500748));
#51280=DIRECTION('',(0.,-0.999960936647921,0.00883884484604973));
#51281=DIRECTION('center_axis',(1.,0.,0.));
#51282=DIRECTION('ref_axis',(0.,-0.500000000000001,0.866025403784438));
#51283=DIRECTION('',(0.,-0.492325804147173,-0.870410996352206));
#51284=DIRECTION('',(0.,-0.870410996352206,-0.492325804147173));
#51285=DIRECTION('center_axis',(1.,0.,0.));
#51286=DIRECTION('ref_axis',(0.,-0.866025403784441,0.499999999999996));
#51287=DIRECTION('',(0.,0.00883884484605022,-0.999960936647921));
#51288=DIRECTION('',(0.,-0.507635132500748,-0.861572151506157));
#51289=DIRECTION('center_axis',(1.,0.,0.));
#51290=DIRECTION('ref_axis',(0.,-1.,0.));
#51291=DIRECTION('',(0.,0.507635132500748,-0.861572151506157));
#51292=DIRECTION('',(0.,-0.00883884484604923,-0.999960936647921));
#51293=DIRECTION('center_axis',(1.,0.,0.));
#51294=DIRECTION('ref_axis',(0.,-0.866025403784436,-0.500000000000004));
#51295=DIRECTION('',(0.,0.870410996352206,-0.492325804147172));
#51296=DIRECTION('',(0.,0.492325804147172,-0.870410996352206));
#51297=DIRECTION('center_axis',(1.,0.,0.));
#51298=DIRECTION('ref_axis',(0.,-0.500000000000001,-0.866025403784438));
#51299=DIRECTION('',(0.,0.999960936647921,0.00883884484604825));
#51300=DIRECTION('',(0.,0.861572151506156,-0.507635132500749));
#51301=DIRECTION('center_axis',(1.,0.,0.));
#51302=DIRECTION('ref_axis',(0.,-4.53023906834102E-16,-1.));
#51303=DIRECTION('',(0.,0.861572151506157,0.507635132500748));
#51304=DIRECTION('',(0.,0.999960936647921,-0.00883884484604873));
#51305=DIRECTION('center_axis',(1.,0.,0.));
#51306=DIRECTION('ref_axis',(0.,0.500000000000001,-0.866025403784438));
#51307=DIRECTION('',(0.,0.492325804147172,0.870410996352206));
#51308=DIRECTION('',(0.,0.870410996352206,0.492325804147172));
#51309=DIRECTION('center_axis',(1.,0.,0.));
#51310=DIRECTION('ref_axis',(0.,0.866025403784438,-0.500000000000001));
#51311=DIRECTION('center_axis',(0.161706903632284,-0.878723185949186,-0.449106267817508));
#51312=DIRECTION('ref_axis',(-0.297687336141045,-0.477331711156208,0.826762775786341));
#51313=DIRECTION('center_axis',(-1.,3.78399284845364E-16,2.07840474806E-15));
#51314=DIRECTION('ref_axis',(1.38777878078144E-15,-0.870410996352205,0.492325804147174));
#51315=DIRECTION('center_axis',(0.413542145111137,-0.91044941088483,0.0080476354506054));
#51316=DIRECTION('ref_axis',(-0.745241313525098,-0.333397429734914,0.577461287413745));
#51317=DIRECTION('center_axis',(0.413542145111137,0.448255248701795,0.792496136412142));
#51318=DIRECTION('ref_axis',(-0.745241313525099,-0.333397429734913,0.577461287413744));
#51319=DIRECTION('center_axis',(1.,0.,0.));
#51320=DIRECTION('ref_axis',(0.,-0.500000000000001,0.866025403784438));
#51321=DIRECTION('',(1.,0.,0.));
#51322=DIRECTION('',(-1.,0.,0.));
#51323=DIRECTION('center_axis',(0.,-0.870410996352206,0.492325804147173));
#51324=DIRECTION('ref_axis',(0.,-0.492325804147173,-0.870410996352206));
#51325=DIRECTION('',(0.,-0.492325804147173,-0.870410996352206));
#51326=DIRECTION('center_axis',(0.,0.870410996352206,-0.492325804147173));
#51327=DIRECTION('ref_axis',(0.,0.492325804147173,0.870410996352206));
#51328=DIRECTION('',(1.,0.,0.));
#51329=DIRECTION('center_axis',(1.,0.,0.));
#51330=DIRECTION('ref_axis',(0.,0.,-1.));
#51331=DIRECTION('center_axis',(-1.,0.,0.));
#51332=DIRECTION('ref_axis',(0.,-1.,1.83697019872103E-16));
#51333=DIRECTION('center_axis',(0.,-1.,-1.22464679914735E-16));
#51334=DIRECTION('ref_axis',(0.,-1.22464679914735E-16,1.));
#51335=DIRECTION('center_axis',(1.,0.,0.));
#51336=DIRECTION('ref_axis',(0.,0.,-1.));
#51337=DIRECTION('center_axis',(1.,0.,0.));
#51338=DIRECTION('ref_axis',(0.,-1.,1.83697019872103E-16));
#51339=DIRECTION('center_axis',(1.,0.,0.));
#51340=DIRECTION('ref_axis',(0.,0.,-1.));
#51341=DIRECTION('center_axis',(-1.,0.,0.));
#51342=DIRECTION('ref_axis',(0.,-1.,1.83697019872103E-16));
#51343=DIRECTION('center_axis',(-1.,0.,0.));
#51344=DIRECTION('ref_axis',(0.,-1.,1.83697019872103E-16));
#51345=DIRECTION('center_axis',(0.,-1.,-1.22464679914735E-16));
#51346=DIRECTION('ref_axis',(0.,-1.22464679914735E-16,1.));
#51347=DIRECTION('center_axis',(1.,0.,0.));
#51348=DIRECTION('ref_axis',(0.,1.,0.));
#51349=DIRECTION('',(-1.,0.,0.));
#51350=DIRECTION('center_axis',(1.,0.,0.));
#51351=DIRECTION('ref_axis',(0.,-1.,1.83697019872103E-16));
#51352=DIRECTION('center_axis',(1.,0.,0.));
#51353=DIRECTION('ref_axis',(0.,-1.,1.83697019872103E-16));
#51354=DIRECTION('center_axis',(1.,0.,0.));
#51355=DIRECTION('ref_axis',(0.,0.,-1.));
#51356=DIRECTION('center_axis',(-1.,0.,0.));
#51357=DIRECTION('ref_axis',(0.,-1.,3.06161699786838E-17));
#51358=DIRECTION('center_axis',(-1.,0.,0.));
#51359=DIRECTION('ref_axis',(0.,-1.,3.06161699786838E-17));
#51360=DIRECTION('center_axis',(0.,-1.,-1.22464679914735E-16));
#51361=DIRECTION('ref_axis',(0.,-1.22464679914735E-16,1.));
#51362=DIRECTION('center_axis',(-1.,0.,0.));
#51363=DIRECTION('ref_axis',(0.,1.,0.));
#51364=DIRECTION('center_axis',(1.,0.,0.));
#51365=DIRECTION('ref_axis',(0.,1.,6.12323399573676E-17));
#51366=DIRECTION('',(0.668964731622449,0.743294146247167,9.10272797026557E-17));
#51367=DIRECTION('center_axis',(1.,0.,0.));
#51368=DIRECTION('ref_axis',(0.,1.,6.12323399573676E-17));
#51369=DIRECTION('center_axis',(1.,0.,0.));
#51370=DIRECTION('ref_axis',(0.,-0.866025403784441,0.499999999999996));
#51371=DIRECTION('center_axis',(1.,0.,0.));
#51372=DIRECTION('ref_axis',(0.,-0.492325804147173,0.870410996352206));
#51373=DIRECTION('',(1.,0.,0.));
#51374=DIRECTION('',(-1.,0.,0.));
#51375=DIRECTION('center_axis',(-0.413542145111131,0.792496136412145,0.448255248701794));
#51376=DIRECTION('ref_axis',(-0.745241313525101,-0.577461287413739,0.333397429734917));
#51377=DIRECTION('center_axis',(0.338418745226395,-0.81905293332663,-0.463276424274359));
#51378=DIRECTION('ref_axis',(0.,-0.492325804147171,0.870410996352207));
#51379=DIRECTION('center_axis',(0.,-0.870410996352206,-0.492325804147173));
#51380=DIRECTION('ref_axis',(-0.707106781186546,-0.348126914665587,0.615473517939986));
#51381=DIRECTION('center_axis',(-1.36647860845322E-15,0.870410996352205,
0.492325804147175));
#51382=DIRECTION('ref_axis',(-1.,0.,-2.77555756156289E-15));
#51383=DIRECTION('',(0.,0.870410996352206,0.492325804147173));
#51384=DIRECTION('',(0.,-0.870410996352206,-0.492325804147173));
#51385=DIRECTION('center_axis',(0.,0.,1.));
#51386=DIRECTION('ref_axis',(1.,0.,0.));
#51387=DIRECTION('center_axis',(0.,0.599112023568166,0.800665212942374));
#51388=DIRECTION('ref_axis',(0.,-0.800665212942374,0.599112023568166));
#51389=DIRECTION('center_axis',(0.,0.,1.));
#51390=DIRECTION('ref_axis',(1.,0.,0.));
#51391=DIRECTION('center_axis',(0.413542145111137,-0.00804763545060584,
0.91044941088483));
#51392=DIRECTION('ref_axis',(-0.745241313525097,-0.577461287413744,0.333397429734916));
#51393=DIRECTION('center_axis',(0.,-0.999960936647921,-0.00883884484605022));
#51394=DIRECTION('ref_axis',(0.,0.00883884484605022,-0.999960936647921));
#51395=DIRECTION('',(0.,-0.00883884484605022,0.999960936647921));
#51396=DIRECTION('',(1.,0.,0.));
#51397=DIRECTION('center_axis',(-0.338418745228229,0.00831731426729575,
-0.940958859441543));
#51398=DIRECTION('ref_axis',(-0.745241313525101,-0.612903724507645,0.262610755872716));
#51399=DIRECTION('center_axis',(1.,0.,0.));
#51400=DIRECTION('ref_axis',(0.,1.,0.));
#51401=DIRECTION('center_axis',(-1.,-8.96736759784938E-18,-1.50724816044729E-17));
#51402=DIRECTION('ref_axis',(0.,-0.859401817746092,0.51130080740667));
#51403=DIRECTION('center_axis',(-1.,0.,0.));
#51404=DIRECTION('ref_axis',(0.,0.,1.));
#51405=DIRECTION('center_axis',(1.,0.,0.));
#51406=DIRECTION('ref_axis',(0.,-0.859401817746092,0.51130080740667));
#51407=DIRECTION('center_axis',(0.,0.393840402550487,0.919178838593922));
#51408=DIRECTION('ref_axis',(-1.,0.,0.));
#51409=DIRECTION('center_axis',(1.,0.,0.));
#51410=DIRECTION('ref_axis',(0.,0.,-1.));
#51411=DIRECTION('center_axis',(1.,0.,0.));
#51412=DIRECTION('ref_axis',(0.,-0.5,0.866025403784438));
#51413=DIRECTION('',(0.,-0.999960936647921,0.00883884484604973));
#51414=DIRECTION('',(0.,-0.861572151506157,-0.507635132500748));
#51415=DIRECTION('center_axis',(1.,0.,0.));
#51416=DIRECTION('ref_axis',(0.,-1.27103528959282E-15,1.));
#51417=DIRECTION('',(0.,-0.861572151506157,0.507635132500748));
#51418=DIRECTION('',(0.,-0.999960936647921,-0.00883884484604923));
#51419=DIRECTION('center_axis',(1.,0.,0.));
#51420=DIRECTION('ref_axis',(0.,0.500000000000001,0.866025403784438));
#51421=DIRECTION('',(0.,-0.492325804147172,0.870410996352206));
#51422=DIRECTION('',(0.,-0.870410996352206,0.492325804147173));
#51423=DIRECTION('center_axis',(1.,0.,0.));
#51424=DIRECTION('ref_axis',(0.,0.866025403784439,0.5));
#51425=DIRECTION('',(0.,0.00883884484604973,0.999960936647921));
#51426=DIRECTION('',(0.,-0.507635132500748,0.861572151506157));
#51427=DIRECTION('center_axis',(1.,0.,0.));
#51428=DIRECTION('ref_axis',(0.,1.,0.));
#51429=DIRECTION('',(0.,0.507635132500748,0.861572151506157));
#51430=DIRECTION('',(0.,-0.00883884484604825,0.999960936647921));
#51431=DIRECTION('center_axis',(1.,0.,0.));
#51432=DIRECTION('ref_axis',(0.,0.866025403784438,-0.5));
#51433=DIRECTION('',(0.,0.870410996352206,0.492325804147172));
#51434=DIRECTION('',(0.,0.492325804147172,0.870410996352206));
#51435=DIRECTION('center_axis',(1.,0.,0.));
#51436=DIRECTION('ref_axis',(0.,0.5,-0.866025403784439));
#51437=DIRECTION('',(0.,0.999960936647921,-0.00883884484604873));
#51438=DIRECTION('',(0.,0.861572151506157,0.507635132500748));
#51439=DIRECTION('center_axis',(1.,0.,0.));
#51440=DIRECTION('ref_axis',(0.,-1.60812264967664E-16,-1.));
#51441=DIRECTION('',(0.,0.861572151506156,-0.507635132500749));
#51442=DIRECTION('',(0.,0.999960936647921,0.00883884484604825));
#51443=DIRECTION('center_axis',(1.,0.,0.));
#51444=DIRECTION('ref_axis',(0.,-0.5,-0.866025403784438));
#51445=DIRECTION('',(0.,0.492325804147172,-0.870410996352206));
#51446=DIRECTION('',(0.,0.870410996352206,-0.492325804147172));
#51447=DIRECTION('center_axis',(1.,0.,0.));
#51448=DIRECTION('ref_axis',(0.,-0.866025403784439,-0.5));
#51449=DIRECTION('',(0.,-0.00883884484604923,-0.999960936647921));
#51450=DIRECTION('',(0.,0.507635132500748,-0.861572151506157));
#51451=DIRECTION('center_axis',(1.,0.,0.));
#51452=DIRECTION('ref_axis',(0.,-1.,-1.22464679914735E-16));
#51453=DIRECTION('',(0.,-0.507635132500748,-0.861572151506157));
#51454=DIRECTION('',(0.,0.00883884484605022,-0.999960936647921));
#51455=DIRECTION('center_axis',(-1.,0.,0.));
#51456=DIRECTION('ref_axis',(0.,1.,0.));
#51457=DIRECTION('center_axis',(0.,0.,1.));
#51458=DIRECTION('ref_axis',(1.,0.,0.));
#51459=DIRECTION('center_axis',(-0.338418745227643,0.477682435167614,0.810735619058942));
#51460=DIRECTION('ref_axis',(-0.745241313525099,-0.662095573434012,0.0790242763615819));
#51461=DIRECTION('center_axis',(0.,-0.507635132500748,-0.861572151506157));
#51462=DIRECTION('ref_axis',(-0.707106781186549,-0.609223510811485,0.358952244559811));
#51463=DIRECTION('center_axis',(0.,0.118513625651546,0.992952426118656));
#51464=DIRECTION('ref_axis',(0.,-0.992952426118656,0.118513625651546));
#51465=DIRECTION('center_axis',(-0.413542145111134,0.462194162183031,0.78444850096154));
#51466=DIRECTION('ref_axis',(-0.745241313525099,-0.666794859469827,-3.46944695195361E-16));
#51467=DIRECTION('center_axis',(0.,0.507635132500748,-0.861572151506157));
#51468=DIRECTION('ref_axis',(-0.707106781186549,-0.609223510811484,-0.358952244559812));
#51469=DIRECTION('center_axis',(-5.9783577498623E-16,0.507635132500748,
-0.861572151506157));
#51470=DIRECTION('ref_axis',(0.,-0.861572151506157,-0.507635132500748));
#51471=DIRECTION('center_axis',(0.,0.258819045102522,-0.965925826289068));
#51472=DIRECTION('ref_axis',(6.68632116760916E-16,-0.965925826289068,-0.258819045102522));
#51473=DIRECTION('',(0.,-0.507635132500748,0.861572151506157));
#51474=DIRECTION('center_axis',(0.338418745226384,-0.477682435167847,0.810735619059331));
#51475=DIRECTION('ref_axis',(-0.745241313526798,-0.662095573432159,-0.0790242763610905));
#51476=DIRECTION('center_axis',(-0.413542145111139,0.462194162183039,-0.784448500961533));
#51477=DIRECTION('ref_axis',(-1.38777878078145E-15,-0.861572151506154,-0.507635132500752));
#51478=DIRECTION('center_axis',(0.,0.,1.));
#51479=DIRECTION('ref_axis',(1.,0.,0.));
#51480=DIRECTION('center_axis',(0.,0.118513625651149,-0.992952426118704));
#51481=DIRECTION('ref_axis',(0.,-0.992952426118703,-0.118513625651149));
#51482=DIRECTION('center_axis',(0.,0.,1.));
#51483=DIRECTION('ref_axis',(1.,0.,0.));
#51484=DIRECTION('center_axis',(-1.,0.,0.));
#51485=DIRECTION('ref_axis',(0.,-1.,0.));
#51486=DIRECTION('center_axis',(0.,-0.861572151506157,0.507635132500748));
#51487=DIRECTION('ref_axis',(0.,-0.507635132500748,-0.861572151506157));
#51488=DIRECTION('',(-1.,0.,0.));
#51489=DIRECTION('',(0.,0.507635132500748,0.861572151506157));
#51490=DIRECTION('center_axis',(1.,0.,0.));
#51491=DIRECTION('ref_axis',(0.,-1.,0.));
#51492=DIRECTION('',(1.,0.,0.));
#51493=DIRECTION('center_axis',(0.,-0.861572151506157,-0.507635132500748));
#51494=DIRECTION('ref_axis',(0.,0.507635132500748,-0.861572151506157));
#51495=DIRECTION('',(1.,0.,0.));
#51496=DIRECTION('center_axis',(0.,-0.00883884484604825,0.999960936647921));
#51497=DIRECTION('ref_axis',(-0.70710678118655,0.707079159225394,0.00625000712849673));
#51498=DIRECTION('center_axis',(0.,-0.00883884484604859,0.999960936647921));
#51499=DIRECTION('ref_axis',(0.,0.999960936647921,0.00883884484604859));
#51500=DIRECTION('center_axis',(0.,-0.861572151506157,0.507635132500748));
#51501=DIRECTION('ref_axis',(4.46891313140503E-17,0.507635132500748,0.861572151506157));
#51502=DIRECTION('',(0.,0.00883884484604825,-0.999960936647921));
#51503=DIRECTION('center_axis',(0.338418745226294,0.00831731426730007,-0.940958859442239));
#51504=DIRECTION('ref_axis',(-0.745241313526918,0.612903724505889,-0.262610755871659));
#51505=DIRECTION('center_axis',(-0.413542145111135,-0.00804763545060408,
0.910449410884831));
#51506=DIRECTION('ref_axis',(6.93889390390723E-16,0.999960936647921,0.00883884484604859));
#51507=DIRECTION('center_axis',(0.,0.,1.));
#51508=DIRECTION('ref_axis',(1.,0.,0.));
#51509=DIRECTION('center_axis',(0.,0.393840402550884,0.919178838593751));
#51510=DIRECTION('ref_axis',(0.,0.919178838593751,-0.393840402550884));
#51511=DIRECTION('center_axis',(1.,0.,0.));
#51512=DIRECTION('ref_axis',(0.,0.866025403784438,-0.500000000000001));
#51513=DIRECTION('center_axis',(1.,0.,0.));
#51514=DIRECTION('ref_axis',(0.,0.492325804147172,-0.870410996352206));
#51515=DIRECTION('',(1.,0.,0.));
#51516=DIRECTION('',(-1.,0.,0.));
#51517=DIRECTION('center_axis',(0.,0.,1.));
#51518=DIRECTION('ref_axis',(1.,0.,0.));
#51519=DIRECTION('center_axis',(0.413542145111137,0.792496136412142,0.448255248701794));
#51520=DIRECTION('ref_axis',(-0.745241313525094,0.577461287413753,-0.333397429734907));
#51521=DIRECTION('center_axis',(-1.,0.,0.));
#51522=DIRECTION('ref_axis',(0.,0.,1.));
#51523=DIRECTION('center_axis',(-1.,2.67375340674029E-17,2.00032569009636E-17));
#51524=DIRECTION('ref_axis',(1.3153755286441E-17,0.866025403784438,-0.5));
#51525=DIRECTION('center_axis',(0.,-0.599112023568166,-0.800665212942374));
#51526=DIRECTION('ref_axis',(0.,0.800665212942374,-0.599112023568166));
#51527=DIRECTION('center_axis',(1.,0.,0.));
#51528=DIRECTION('ref_axis',(0.,1.,0.));
#51529=DIRECTION('center_axis',(0.338418745226028,0.819052933326745,0.463276424274424));
#51530=DIRECTION('ref_axis',(6.93889390390724E-16,0.492325804147171,-0.870410996352207));
#51531=DIRECTION('center_axis',(0.,0.492325804147172,-0.870410996352206));
#51532=DIRECTION('ref_axis',(0.,0.870410996352206,0.492325804147172));
#51533=DIRECTION('',(1.,0.,0.));
#51534=DIRECTION('',(0.,-0.870410996352206,-0.492325804147172));
#51535=DIRECTION('center_axis',(1.,0.,0.));
#51536=DIRECTION('ref_axis',(0.,-0.866025403784436,-0.500000000000004));
#51537=DIRECTION('',(1.,0.,0.));
#51538=DIRECTION('',(-1.,0.,0.));
#51539=DIRECTION('center_axis',(0.338418745226007,-0.00831731426730377,
-0.940958859442343));
#51540=DIRECTION('ref_axis',(3.46944695195362E-16,-0.999960936647921,0.00883884484605136));
#51541=DIRECTION('center_axis',(0.,-0.00883884484604923,-0.999960936647921));
#51542=DIRECTION('ref_axis',(-0.70710678118655,-0.707079159225394,0.00625000712849772));
#51543=DIRECTION('center_axis',(-4.90654452958627E-17,0.00883884484604859,
0.999960936647921));
#51544=DIRECTION('ref_axis',(-1.,-5.55111512312578E-15,0.));
#51545=DIRECTION('',(0.,0.00883884484604923,0.999960936647921));
#51546=DIRECTION('center_axis',(0.,0.,1.));
#51547=DIRECTION('ref_axis',(1.,0.,0.));
#51548=DIRECTION('center_axis',(0.,-0.39384040255049,0.91917883859392));
#51549=DIRECTION('ref_axis',(0.,-0.91917883859392,-0.39384040255049));
#51550=DIRECTION('center_axis',(0.,-0.492325804147172,-0.870410996352206));
#51551=DIRECTION('ref_axis',(0.,0.870410996352206,-0.492325804147172));
#51552=DIRECTION('',(0.,-0.870410996352206,0.492325804147172));
#51553=DIRECTION('',(1.,0.,0.));
#51554=DIRECTION('center_axis',(1.,0.,0.));
#51555=DIRECTION('ref_axis',(0.,1.,0.));
#51556=DIRECTION('center_axis',(-1.,4.3002349452093E-19,2.55626880319234E-17));
#51557=DIRECTION('ref_axis',(-1.3153755286441E-17,-0.866025403784439,-0.5));
#51558=DIRECTION('center_axis',(-1.,0.,0.));
#51559=DIRECTION('ref_axis',(0.,0.,1.));
#51560=DIRECTION('center_axis',(1.,0.,0.));
#51561=DIRECTION('ref_axis',(0.,-1.,1.99962609112443E-13));
#51562=DIRECTION('center_axis',(-1.,0.,0.));
#51563=DIRECTION('ref_axis',(0.,-1.,-1.22464679914735E-16));
#51564=DIRECTION('center_axis',(0.,-0.507635132500748,-0.861572151506157));
#51565=DIRECTION('ref_axis',(-0.707106781186549,-0.609223510811484,0.358952244559812));
#51566=DIRECTION('center_axis',(0.,0.258819045102523,0.965925826289068));
#51567=DIRECTION('ref_axis',(-1.83873832109252E-15,-0.965925826289068,0.258819045102523));
#51568=DIRECTION('center_axis',(-1.,0.,0.));
#51569=DIRECTION('ref_axis',(0.,0.,1.));
#51570=DIRECTION('center_axis',(0.,0.870410996352206,-0.492325804147172));
#51571=DIRECTION('ref_axis',(-0.707106781186551,-0.348126914665582,-0.615473517939983));
#51572=DIRECTION('center_axis',(0.,0.707106781186545,-0.70710678118655));
#51573=DIRECTION('ref_axis',(2.3402124086632E-15,-0.70710678118655,-0.707106781186545));
#51574=DIRECTION('center_axis',(0.,-0.999960936647921,0.00883884484604923));
#51575=DIRECTION('ref_axis',(0.,-0.00883884484604923,-0.999960936647921));
#51576=DIRECTION('center_axis',(0.,0.492325804147172,0.870410996352206));
#51577=DIRECTION('ref_axis',(-0.707106781186551,0.615473517939983,-0.348126914665582));
#51578=DIRECTION('',(0.,-0.492325804147172,-0.870410996352206));
#51579=DIRECTION('center_axis',(0.,0.492325804147173,0.870410996352206));
#51580=DIRECTION('ref_axis',(0.,0.870410996352206,-0.492325804147173));
#51581=DIRECTION('center_axis',(0.,-0.70710678118655,-0.707106781186545));
#51582=DIRECTION('ref_axis',(0.,0.707106781186545,-0.70710678118655));
#51583=DIRECTION('center_axis',(0.,0.870410996352206,0.492325804147172));
#51584=DIRECTION('ref_axis',(-0.707106781186546,0.348126914665583,-0.615473517939987));
#51585=DIRECTION('center_axis',(-1.36647860845322E-15,-0.870410996352205,
-0.492325804147175));
#51586=DIRECTION('ref_axis',(-1.,0.,2.77555756156289E-15));
#51587=DIRECTION('center_axis',(0.338418745226388,-0.46327642427436,-0.819052933326632));
#51588=DIRECTION('ref_axis',(-0.745241313526793,0.399484817560469,-0.533879448144934));
#51589=DIRECTION('center_axis',(-0.413542145111136,0.448255248701793,0.792496136412142));
#51590=DIRECTION('ref_axis',(6.93889390390724E-16,0.870410996352207,-0.492325804147171));
#51591=DIRECTION('center_axis',(-0.161706903632285,-0.878723185949184,-0.449106267817512));
#51592=DIRECTION('ref_axis',(-0.297687336141044,0.477331711156212,-0.826762775786339));
#51593=DIRECTION('center_axis',(-1.,0.,0.));
#51594=DIRECTION('ref_axis',(0.,0.500000000000001,-0.866025403784438));
#51595=DIRECTION('center_axis',(0.413542145111136,0.91044941088483,-0.00804763545060449));
#51596=DIRECTION('ref_axis',(-0.745241313525101,0.333397429734915,-0.577461287413741));
#51597=DIRECTION('center_axis',(0.,0.,1.));
#51598=DIRECTION('ref_axis',(1.,0.,0.));
#51599=DIRECTION('center_axis',(0.,0.800665212942613,0.599112023567847));
#51600=DIRECTION('ref_axis',(0.,0.599112023567847,-0.800665212942613));
#51601=DIRECTION('center_axis',(0.,0.,1.));
#51602=DIRECTION('ref_axis',(1.,0.,0.));
#51603=DIRECTION('center_axis',(0.,0.999960936647921,0.00883884484604825));
#51604=DIRECTION('ref_axis',(0.,-0.00883884484604825,0.999960936647921));
#51605=DIRECTION('',(1.,0.,0.));
#51606=DIRECTION('center_axis',(-1.,0.,0.));
#51607=DIRECTION('ref_axis',(0.,0.,1.));
#51608=DIRECTION('center_axis',(-1.,9.62921718000255E-18,3.59367277528846E-17));
#51609=DIRECTION('ref_axis',(-2.6307510572882E-17,0.5,-0.866025403784439));
#51610=DIRECTION('center_axis',(0.,-0.91917883859392,-0.39384040255049));
#51611=DIRECTION('ref_axis',(0.,0.39384040255049,-0.91917883859392));
#51612=DIRECTION('center_axis',(1.,0.,0.));
#51613=DIRECTION('ref_axis',(0.,1.,0.));
#51614=DIRECTION('center_axis',(1.,0.,0.));
#51615=DIRECTION('ref_axis',(0.,0.500000000000001,-0.866025403784438));
#51616=DIRECTION('',(1.,0.,0.));
#51617=DIRECTION('',(-1.,0.,0.));
#51618=DIRECTION('center_axis',(0.338418745226014,0.94095885944234,-0.0083173142673009));
#51619=DIRECTION('ref_axis',(1.04083408558609E-15,-0.00883884484604859,
-0.999960936647921));
#51620=DIRECTION('center_axis',(0.,0.861572151506157,0.507635132500748));
#51621=DIRECTION('ref_axis',(-0.70710678118655,0.358952244559809,-0.609223510811485));
#51622=DIRECTION('',(0.,-0.861572151506157,-0.507635132500748));
#51623=DIRECTION('center_axis',(1.19567154997246E-15,0.861572151506157,
0.507635132500748));
#51624=DIRECTION('ref_axis',(0.,0.507635132500748,-0.861572151506157));
#51625=DIRECTION('center_axis',(1.34049136553276E-15,-0.965925826289071,
-0.25881904510251));
#51626=DIRECTION('ref_axis',(-4.83154842407171E-15,0.25881904510251,-0.965925826289071));
#51627=DIRECTION('center_axis',(0.,0.999960936647921,-0.00883884484604873));
#51628=DIRECTION('ref_axis',(-0.707106781186546,-0.0062500071284967,-0.707079159225398));
#51629=DIRECTION('center_axis',(0.,-0.999960936647921,0.00883884484604859));
#51630=DIRECTION('ref_axis',(-1.,0.,0.));
#51631=DIRECTION('',(0.,-0.999960936647921,0.00883884484604873));
#51632=DIRECTION('center_axis',(1.33226762955019E-14,-1.,4.44089209850062E-14));
#51633=DIRECTION('ref_axis',(-0.297687338842933,-4.46251367491381E-14,-0.954663421469898));
#51634=DIRECTION('center_axis',(0.413542156800177,-0.784448496387312,-0.462194159487918));
#51635=DIRECTION('ref_axis',(6.93889390390723E-16,0.507635132500748,-0.861572151506157));
#51636=DIRECTION('center_axis',(-1.,-7.31019564161356E-9,4.30714029771003E-9));
#51637=DIRECTION('ref_axis',(0.,-0.507635132500749,-0.861572151506156));
#51638=DIRECTION('center_axis',(0.413542145111231,0.784448500961426,-0.462194162183139));
#51639=DIRECTION('ref_axis',(-0.745241313525099,6.93889390390722E-16,-0.666794859469826));
#51640=DIRECTION('center_axis',(1.,0.,0.));
#51641=DIRECTION('ref_axis',(0.,-4.53023906834102E-16,-1.));
#51642=DIRECTION('',(-1.,0.,0.));
#51643=DIRECTION('',(1.,0.,0.));
#51644=DIRECTION('center_axis',(0.338418745226036,0.81073561905944,-0.477682435167908));
#51645=DIRECTION('ref_axis',(0.,-0.507635132500748,-0.861572151506157));
#51646=DIRECTION('center_axis',(0.338418745226025,-0.810735619059443,-0.47768243516791));
#51647=DIRECTION('ref_axis',(-0.745241313527275,0.079024276360955,-0.662095573431637));
#51648=DIRECTION('center_axis',(0.,0.999960936647921,0.00883884484604825));
#51649=DIRECTION('ref_axis',(-0.70710678118655,0.00625000712849673,-0.707079159225394));
#51650=DIRECTION('',(0.,-0.999960936647921,-0.00883884484604825));
#51651=DIRECTION('center_axis',(2.77544913898065E-15,0.999960936647921,
0.00883884484604859));
#51652=DIRECTION('ref_axis',(0.,0.00883884484604859,-0.999960936647921));
#51653=DIRECTION('center_axis',(-1.34049136553275E-15,-0.965925826289069,
0.258819045102519));
#51654=DIRECTION('ref_axis',(4.83154842407195E-15,-0.258819045102519,-0.965925826289069));
#51655=DIRECTION('center_axis',(0.,0.861572151506156,-0.507635132500749));
#51656=DIRECTION('ref_axis',(-0.707106781186549,-0.358952244559813,-0.609223510811484));
#51657=DIRECTION('center_axis',(1.96474513883499E-15,-0.861572151506157,
0.507635132500747));
#51658=DIRECTION('ref_axis',(-1.,-5.55111512312578E-15,-5.55111512312578E-15));
#51659=DIRECTION('',(0.,-0.861572151506156,0.507635132500749));
#51660=DIRECTION('center_axis',(0.161706903632265,-0.878723185949164,0.449106267817557));
#51661=DIRECTION('ref_axis',(-0.297687336140981,-0.477331711156245,-0.826762775786342));
#51662=DIRECTION('center_axis',(0.413542145111141,-0.910449410884828,-0.00804763545060434));
#51663=DIRECTION('ref_axis',(0.,0.00883884484604859,-0.999960936647921));
#51664=DIRECTION('center_axis',(-1.,4.41314269147647E-14,-7.80224780983495E-14));
#51665=DIRECTION('ref_axis',(0.,-0.870410996352207,-0.492325804147171));
#51666=DIRECTION('center_axis',(0.413542145111205,0.44825524870168,-0.792496136412171));
#51667=DIRECTION('ref_axis',(-0.745241313525101,-0.333397429734915,-0.57746128741374));
#51668=DIRECTION('center_axis',(1.,0.,0.));
#51669=DIRECTION('ref_axis',(0.,-0.500000000000001,-0.866025403784438));
#51670=DIRECTION('',(-1.,0.,0.));
#51671=DIRECTION('',(1.,0.,0.));
#51672=DIRECTION('center_axis',(0.338418745226017,0.463276424274426,-0.819052933326748));
#51673=DIRECTION('ref_axis',(3.46944695195362E-16,-0.870410996352207,-0.492325804147171));
#51674=DIRECTION('center_axis',(0.338418745226013,-0.94095885944234,-0.00831731426729853));
#51675=DIRECTION('ref_axis',(-0.745241313527289,-0.262610755871546,-0.612903724505486));
#51676=DIRECTION('center_axis',(0.,0.492325804147172,-0.870410996352206));
#51677=DIRECTION('ref_axis',(-0.707106781186546,-0.615473517939987,-0.348126914665583));
#51678=DIRECTION('center_axis',(4.83175164518571E-15,-0.492325804147171,
0.870410996352207));
#51679=DIRECTION('ref_axis',(-1.,0.,5.55111512312578E-15));
#51680=DIRECTION('',(0.,-0.492325804147172,0.870410996352206));
#51681=DIRECTION('center_axis',(0.,0.,1.));
#51682=DIRECTION('ref_axis',(1.,0.,0.));
#51683=DIRECTION('center_axis',(0.,-0.800665212942374,0.599112023568166));
#51684=DIRECTION('ref_axis',(0.,-0.599112023568166,-0.800665212942374));
#51685=DIRECTION('center_axis',(1.,0.,0.));
#51686=DIRECTION('ref_axis',(0.,-1.,0.));
#51687=DIRECTION('center_axis',(0.,0.919178838593717,-0.393840402550966));
#51688=DIRECTION('ref_axis',(0.,-0.393840402550966,-0.919178838593716));
#51689=DIRECTION('center_axis',(0.,0.,1.));
#51690=DIRECTION('ref_axis',(1.,0.,0.));
#51691=DIRECTION('center_axis',(0.,-0.992952426118656,0.118513625651547));
#51692=DIRECTION('ref_axis',(0.,-0.118513625651547,-0.992952426118656));
#51693=DIRECTION('center_axis',(0.,0.,1.));
#51694=DIRECTION('ref_axis',(1.,0.,0.));
#51695=DIRECTION('center_axis',(0.,0.992952426118717,0.118513625651036));
#51696=DIRECTION('ref_axis',(0.,0.118513625651036,-0.992952426118717));
#51697=DIRECTION('center_axis',(1.,0.,0.));
#51698=DIRECTION('ref_axis',(0.,-1.,0.));
#51699=DIRECTION('center_axis',(0.,0.870410996352206,-0.492325804147172));
#51700=DIRECTION('ref_axis',(0.,0.492325804147172,0.870410996352206));
#51701=DIRECTION('center_axis',(1.,0.,0.));
#51702=DIRECTION('ref_axis',(0.,1.,0.));
#51703=DIRECTION('center_axis',(-1.,0.,0.));
#51704=DIRECTION('ref_axis',(0.,-1.11022302462516E-16,-1.));
#51705=DIRECTION('center_axis',(-1.,0.,0.));
#51706=DIRECTION('ref_axis',(0.,1.22464679914735E-16,-1.));
#51707=DIRECTION('center_axis',(1.,0.,0.));
#51708=DIRECTION('ref_axis',(0.,1.,0.));
#51709=DIRECTION('center_axis',(-1.,-1.0804063215482E-17,1.63634943464419E-17));
#51710=DIRECTION('ref_axis',(-8.76917019096067E-18,-0.5,-0.866025403784439));
#51711=DIRECTION('center_axis',(-1.,0.,0.));
#51712=DIRECTION('ref_axis',(0.,0.,1.));
#51713=DIRECTION('center_axis',(0.,-0.870410996352206,-0.492325804147172));
#51714=DIRECTION('ref_axis',(0.,0.492325804147172,-0.870410996352206));
#51715=DIRECTION('center_axis',(0.,-0.507635132500749,-0.861572151506156));
#51716=DIRECTION('ref_axis',(0.,0.861572151506156,-0.507635132500749));
#51717=DIRECTION('',(1.,0.,0.));
#51718=DIRECTION('center_axis',(0.,-0.00883884484604873,-0.999960936647921));
#51719=DIRECTION('ref_axis',(0.,0.999960936647921,-0.00883884484604873));
#51720=DIRECTION('',(1.,0.,0.));
#51721=DIRECTION('center_axis',(0.,0.00883884484605022,-0.999960936647921));
#51722=DIRECTION('ref_axis',(-0.70710678118655,-0.707079159225394,-0.0062500071284987));
#51723=DIRECTION('center_axis',(0.,0.00883884484605141,-0.999960936647921));
#51724=DIRECTION('ref_axis',(7.38853422888047E-12,-0.999960936647921,-0.00883884484605141));
#51725=DIRECTION('center_axis',(0.,0.,1.));
#51726=DIRECTION('ref_axis',(1.,0.,0.));
#51727=DIRECTION('center_axis',(1.,0.,0.));
#51728=DIRECTION('ref_axis',(0.,0.,-1.));
#51729=DIRECTION('center_axis',(0.,-1.,-1.22464679914735E-16));
#51730=DIRECTION('ref_axis',(0.,-1.22464679914735E-16,1.));
#51731=DIRECTION('center_axis',(-1.,0.,0.));
#51732=DIRECTION('ref_axis',(0.,0.,1.));
#51733=DIRECTION('center_axis',(-1.,-3.20973906000084E-18,-1.19789092509615E-17));
#51734=DIRECTION('ref_axis',(-8.76917019096067E-18,-0.5,0.866025403784439));
#51735=DIRECTION('center_axis',(0.,0.00883884484604973,0.999960936647921));
#51736=DIRECTION('ref_axis',(0.,-0.999960936647921,0.00883884484604973));
#51737=DIRECTION('',(1.,0.,0.));
#51738=DIRECTION('center_axis',(0.,-0.00883884484604973,-0.999960936647921));
#51739=DIRECTION('ref_axis',(8.93782626281008E-17,-0.999960936647921,0.00883884484604976));
#51740=DIRECTION('center_axis',(1.,0.,0.));
#51741=DIRECTION('ref_axis',(0.,1.,0.));
#51742=DIRECTION('center_axis',(0.,-1.,0.));
#51743=DIRECTION('ref_axis',(-0.297687336141042,4.15762143992418E-16,0.954663422312414));
#51744=DIRECTION('center_axis',(-1.,-2.05035865121992E-15,2.01343958592934E-15));
#51745=DIRECTION('ref_axis',(2.08166817117216E-15,-0.507635132500745,0.861572151506158));
#51746=DIRECTION('center_axis',(0.413542145111137,-0.784448500961537,0.462194162183035));
#51747=DIRECTION('ref_axis',(-0.745241313525099,0.,0.666794859469826));
#51748=DIRECTION('center_axis',(0.413542145111137,0.784448500961537,0.462194162183035));
#51749=DIRECTION('ref_axis',(-0.745241313525095,1.04083408558608E-15,0.666794859469831));
#51750=DIRECTION('center_axis',(1.,0.,0.));
#51751=DIRECTION('ref_axis',(0.,2.51679948241167E-16,1.));
#51752=DIRECTION('',(1.,0.,0.));
#51753=DIRECTION('',(-1.,0.,0.));
#51754=DIRECTION('center_axis',(0.,-0.507635132500748,0.861572151506157));
#51755=DIRECTION('ref_axis',(0.,-0.861572151506157,-0.507635132500748));
#51756=DIRECTION('',(0.,0.861572151506157,0.507635132500748));
#51757=DIRECTION('center_axis',(-0.338418745227643,-0.810735619058942,-0.477682435167614));
#51758=DIRECTION('ref_axis',(-0.745241313525102,-0.0790242763615876,0.662095573434008));
#51759=DIRECTION('center_axis',(-0.338418745227644,0.810735619058941,-0.477682435167615));
#51760=DIRECTION('ref_axis',(-0.745241313525102,0.0790242763615904,0.662095573434008));
#51761=DIRECTION('center_axis',(0.,-0.861572151506157,0.507635132500748));
#51762=DIRECTION('ref_axis',(-0.70710678118655,0.358952244559809,0.609223510811485));
#51763=DIRECTION('center_axis',(0.,0.861572151506156,-0.50763513250075));
#51764=DIRECTION('ref_axis',(-1.,0.,0.));
#51765=DIRECTION('',(0.,0.861572151506157,-0.507635132500748));
#51766=DIRECTION('center_axis',(0.,0.965925826289067,-0.258819045102524));
#51767=DIRECTION('ref_axis',(2.00589635028275E-15,0.258819045102524,0.965925826289067));
#51768=DIRECTION('center_axis',(-1.,0.,0.));
#51769=DIRECTION('ref_axis',(0.,0.,1.));
#51770=DIRECTION('center_axis',(0.,0.992952426118656,0.118513625651546));
#51771=DIRECTION('ref_axis',(-1.,0.,0.));
#51772=DIRECTION('center_axis',(-1.,0.,0.));
#51773=DIRECTION('ref_axis',(0.,-1.22124532708767E-15,1.));
#51774=DIRECTION('center_axis',(0.,-0.992952426118656,0.118513625651544));
#51775=DIRECTION('ref_axis',(-0.745241313525092,0.0790242763615814,0.66209557343402));
#51776=DIRECTION('center_axis',(0.,0.,1.));
#51777=DIRECTION('ref_axis',(-0.707106781194724,0.707106781178371,0.));
#51778=DIRECTION('center_axis',(0.,-0.861572151506157,-0.507635132500748));
#51779=DIRECTION('ref_axis',(-0.707106781186549,-0.358952244559811,0.609223510811485));
#51780=DIRECTION('center_axis',(0.,-0.861572151506157,-0.507635132500748));
#51781=DIRECTION('ref_axis',(7.80157188851054E-12,-0.507635132500748,0.861572151506157));
#51782=DIRECTION('center_axis',(0.,0.,1.));
#51783=DIRECTION('ref_axis',(1.,0.,0.));
#51784=DIRECTION('center_axis',(1.,0.,0.));
#51785=DIRECTION('ref_axis',(0.,1.,0.));
#51786=DIRECTION('center_axis',(0.,0.507635132500748,0.861572151506157));
#51787=DIRECTION('ref_axis',(0.,-0.861572151506157,0.507635132500748));
#51788=DIRECTION('',(1.,0.,0.));
#51789=DIRECTION('center_axis',(0.,0.,1.));
#51790=DIRECTION('ref_axis',(1.,0.,0.));
#51791=DIRECTION('center_axis',(-1.,4.02687917185871E-16,-3.41726441869988E-15));
#51792=DIRECTION('ref_axis',(-1.38777878078144E-15,0.861572151506156,0.50763513250075));
#51793=DIRECTION('center_axis',(0.413542145111137,0.462194162183035,0.784448500961537));
#51794=DIRECTION('ref_axis',(-0.745241313525095,0.666794859469831,2.42861286636752E-15));
#51795=DIRECTION('center_axis',(0.413542145111137,0.462194162183035,-0.784448500961537));
#51796=DIRECTION('ref_axis',(-0.7452413135251,0.666794859469825,1.7347234759768E-15));
#51797=DIRECTION('center_axis',(1.,0.,0.));
#51798=DIRECTION('ref_axis',(0.,1.,-2.51679948241167E-16));
#51799=DIRECTION('',(1.,0.,0.));
#51800=DIRECTION('',(-1.,0.,0.));
#51801=DIRECTION('center_axis',(0.,0.861572151506157,0.507635132500748));
#51802=DIRECTION('ref_axis',(0.,-0.507635132500748,0.861572151506157));
#51803=DIRECTION('',(1.,0.,0.));
#51804=DIRECTION('center_axis',(0.,0.,1.));
#51805=DIRECTION('ref_axis',(1.,0.,0.));
#51806=DIRECTION('center_axis',(-1.,7.01152421001952E-18,7.93231518201485E-16));
#51807=DIRECTION('ref_axis',(2.08166817117217E-15,0.492325804147175,0.870410996352205));
#51808=DIRECTION('center_axis',(0.413542145111137,0.0080476354506054,0.91044941088483));
#51809=DIRECTION('ref_axis',(-0.745241313525099,0.577461287413745,0.333397429734911));
#51810=DIRECTION('center_axis',(0.413542145111137,0.792496136412142,-0.448255248701795));
#51811=DIRECTION('ref_axis',(-0.745241313525099,0.577461287413744,0.333397429734914));
#51812=DIRECTION('center_axis',(1.,0.,0.));
#51813=DIRECTION('ref_axis',(0.,0.866025403784438,0.500000000000001));
#51814=DIRECTION('',(1.,0.,0.));
#51815=DIRECTION('',(-1.,0.,0.));
#51816=DIRECTION('center_axis',(0.,0.492325804147173,0.870410996352206));
#51817=DIRECTION('ref_axis',(0.,-0.870410996352206,0.492325804147173));
#51818=DIRECTION('center_axis',(0.,-0.492325804147173,-0.870410996352206));
#51819=DIRECTION('ref_axis',(8.93782626281008E-17,0.870410996352206,-0.492325804147173));
#51820=DIRECTION('',(1.,0.,0.));
#51821=DIRECTION('center_axis',(-0.161706903632283,-0.878723185949185,0.449106267817511));
#51822=DIRECTION('ref_axis',(-0.297687336141044,0.477331711156208,0.826762775786341));
#51823=DIRECTION('center_axis',(-1.,-3.78399284845376E-16,2.07840474806E-15));
#51824=DIRECTION('ref_axis',(2.08166817117217E-15,-0.00883884484604859,
0.999960936647921));
#51825=DIRECTION('center_axis',(0.413542145111137,-0.448255248701795,0.792496136412142));
#51826=DIRECTION('ref_axis',(-0.745241313525096,0.333397429734913,0.577461287413748));
#51827=DIRECTION('center_axis',(0.413542145111137,0.91044941088483,0.00804763545060495));
#51828=DIRECTION('ref_axis',(-0.745241313525099,0.333397429734918,0.577461287413741));
#51829=DIRECTION('center_axis',(1.,0.,0.));
#51830=DIRECTION('ref_axis',(0.,0.500000000000001,0.866025403784438));
#51831=DIRECTION('',(1.,0.,0.));
#51832=DIRECTION('',(-1.,0.,0.));
#51833=DIRECTION('center_axis',(0.,-0.00883884484604923,0.999960936647921));
#51834=DIRECTION('ref_axis',(0.,-0.999960936647921,-0.00883884484604923));
#51835=DIRECTION('',(0.,0.999960936647921,0.00883884484604923));
#51836=DIRECTION('center_axis',(-0.338418745227644,-0.940958859441754,-0.00831731426729668));
#51837=DIRECTION('ref_axis',(-0.745241313525102,0.262610755872189,0.612903724507869));
#51838=DIRECTION('center_axis',(-0.338418745227644,0.463276424274139,-0.819052933326238));
#51839=DIRECTION('ref_axis',(-0.745241313525099,0.399484817561819,0.533879448146288));
#51840=DIRECTION('center_axis',(0.,-0.492325804147172,0.870410996352206));
#51841=DIRECTION('ref_axis',(-0.707106781186549,0.615473517939981,0.348126914665589));
#51842=DIRECTION('center_axis',(0.,0.492325804147172,-0.870410996352206));
#51843=DIRECTION('ref_axis',(-1.,0.,0.));
#51844=DIRECTION('',(0.,0.492325804147172,-0.870410996352206));
#51845=DIRECTION('center_axis',(-1.,0.,0.));
#51846=DIRECTION('ref_axis',(0.,0.,1.));
#51847=DIRECTION('center_axis',(0.,0.919178838593919,-0.393840402550494));
#51848=DIRECTION('ref_axis',(-1.,0.,0.));
#51849=DIRECTION('center_axis',(-1.,2.3957818501923E-17,6.41947812000165E-18));
#51850=DIRECTION('ref_axis',(1.75383403819213E-17,0.500000000000001,0.866025403784438));
#51851=DIRECTION('center_axis',(0.,-0.800665212942374,0.599112023568166));
#51852=DIRECTION('ref_axis',(-0.74524131352509,0.399484817561824,0.533879448146297));
#51853=DIRECTION('center_axis',(0.,0.,1.));
#51854=DIRECTION('ref_axis',(1.,0.,0.));
#51855=DIRECTION('center_axis',(0.,-0.999960936647921,-0.00883884484604923));
#51856=DIRECTION('ref_axis',(-0.70710678118655,-0.00625000712849673,0.707079159225394));
#51857=DIRECTION('center_axis',(0.,-0.999960936647921,-0.00883884484604859));
#51858=DIRECTION('ref_axis',(7.38784033949003E-12,-0.00883884484604859,
0.999960936647921));
#51859=DIRECTION('center_axis',(1.,0.,0.));
#51860=DIRECTION('ref_axis',(0.,-1.,0.));
#51861=DIRECTION('center_axis',(1.,0.,0.));
#51862=DIRECTION('ref_axis',(0.,1.,0.));
#51863=DIRECTION('center_axis',(0.,0.870410996352206,0.492325804147172));
#51864=DIRECTION('ref_axis',(0.,-0.492325804147172,0.870410996352206));
#51865=DIRECTION('center_axis',(-1.,0.,0.));
#51866=DIRECTION('ref_axis',(0.,0.,1.));
#51867=DIRECTION('center_axis',(-1.,4.38458509548033E-18,-7.59432415548118E-18));
#51868=DIRECTION('ref_axis',(0.,0.866025403784439,0.5));
#51869=DIRECTION('center_axis',(0.,0.999960936647921,-0.00883884484604973));
#51870=DIRECTION('ref_axis',(0.,0.00883884484604973,0.999960936647921));
#51871=DIRECTION('center_axis',(1.,0.,0.));
#51872=DIRECTION('ref_axis',(0.,1.,0.));
#51873=DIRECTION('center_axis',(-1.,0.,0.));
#51874=DIRECTION('ref_axis',(0.,0.,1.));
#51875=DIRECTION('center_axis',(-1.,0.,0.));
#51876=DIRECTION('ref_axis',(0.,1.,6.12323399573677E-17));
#51877=DIRECTION('center_axis',(0.,0.861572151506157,-0.507635132500748));
#51878=DIRECTION('ref_axis',(0.,0.507635132500748,0.861572151506157));
#51879=DIRECTION('center_axis',(1.,0.,0.));
#51880=DIRECTION('ref_axis',(0.,1.,0.));
#51881=DIRECTION('center_axis',(0.,-0.492325804147173,0.870410996352206));
#51882=DIRECTION('ref_axis',(0.,-0.870410996352206,-0.492325804147173));
#51883=DIRECTION('center_axis',(0.,0.507635132500748,-0.861572151506157));
#51884=DIRECTION('ref_axis',(0.,0.861572151506157,0.507635132500748));
#51885=DIRECTION('center_axis',(0.,0.00883884484604825,-0.999960936647921));
#51886=DIRECTION('ref_axis',(0.,0.999960936647921,0.00883884484604825));
#77126=CARTESIAN_POINT('',(0.,0.,0.));
#77127=CARTESIAN_POINT('Origin',(18.4343145750508,0.,0.));
#77128=CARTESIAN_POINT('',(18.7171572875254,-2.19001660874876E-15,17.8828427124746));
#77129=CARTESIAN_POINT('',(18.7171572875254,-17.8828427124746,-2.19001660874876E-15));
#77130=CARTESIAN_POINT('Origin',(18.7171572875254,0.,-2.73752076093595E-15));
#77131=CARTESIAN_POINT('Origin',(18.7171572875254,0.,-2.73752076093595E-15));
#77132=CARTESIAN_POINT('',(18.4343145750508,-2.20436423846524E-15,18.));
#77133=CARTESIAN_POINT('Origin',(18.4343145750508,-2.15537836649934E-15,
17.6));
#77134=CARTESIAN_POINT('',(18.4343145750508,-18.,-2.20436423846524E-15));
#77135=CARTESIAN_POINT('Origin',(18.4343145750508,0.,0.));
#77136=CARTESIAN_POINT('Origin',(18.4343145750508,0.,0.));
#77137=CARTESIAN_POINT('Origin',(16.8,0.,0.));
#77138=CARTESIAN_POINT('',(15.4,-18.,-2.20436423846524E-15));
#77139=CARTESIAN_POINT('',(16.8,-18.,-2.20436423846524E-15));
#77140=CARTESIAN_POINT('',(15.4,-2.20436423846524E-15,18.));
#77141=CARTESIAN_POINT('Origin',(15.4,0.,0.));
#77142=CARTESIAN_POINT('Origin',(15.4,0.,0.));
#77143=CARTESIAN_POINT('Origin',(18.8,0.,0.));
#77144=CARTESIAN_POINT('',(18.8828427124746,-17.7171572875254,-2.16972599621582E-15));
#77145=CARTESIAN_POINT('',(18.8828427124746,-2.16972599621582E-15,17.7171572875254));
#77146=CARTESIAN_POINT('Origin',(18.8828427124746,0.,-2.71215749526977E-15));
#77147=CARTESIAN_POINT('',(18.8,-17.8,-2.17987130248229E-15));
#77148=CARTESIAN_POINT('Origin',(18.8828427124746,0.,-2.71215749526977E-15));
#77149=CARTESIAN_POINT('Origin',(15.4,0.,0.));
#77150=CARTESIAN_POINT('',(15.,-2.15537836649934E-15,17.6));
#77151=CARTESIAN_POINT('Origin',(15.4,-2.15537836649934E-15,17.6));
#77152=CARTESIAN_POINT('Origin',(15.,0.,0.));
#77153=CARTESIAN_POINT('Origin',(15.,18.,0.));
#77154=CARTESIAN_POINT('',(15.,14.7203487384281,-8.26433068237712));
#77155=CARTESIAN_POINT('',(15.,14.6820725595938,-3.93404948555831));
#77156=CARTESIAN_POINT('',(15.,14.7224318643355,-8.50000000000001));
#77157=CARTESIAN_POINT('',(15.,16.8803613012335,-0.203054053000301));
#77158=CARTESIAN_POINT('',(15.,14.6820725595938,-3.93404948555831));
#77159=CARTESIAN_POINT('',(15.,16.8803613012335,0.2030540530003));
#77160=CARTESIAN_POINT('Origin',(15.,16.5357324406311,2.77555756156289E-16));
#77161=CARTESIAN_POINT('',(15.,14.6820725595938,3.93404948555832));
#77162=CARTESIAN_POINT('',(15.,17.,0.));
#77163=CARTESIAN_POINT('',(15.,14.7203487384281,8.26433068237712));
#77164=CARTESIAN_POINT('',(15.,14.6820725595938,3.93404948555832));
#77165=CARTESIAN_POINT('',(15.,14.5172946854278,8.61603061885642));
#77166=CARTESIAN_POINT('Origin',(15.,14.320364363769,8.26786622031553));
#77167=CARTESIAN_POINT('',(15.,10.7480230740355,10.7480230740355));
#77168=CARTESIAN_POINT('',(15.,14.7224318643355,8.5));
#77169=CARTESIAN_POINT('',(15.,8.61603061885642,14.5172946854278));
#77170=CARTESIAN_POINT('',(15.,10.7480230740355,10.7480230740355));
#77171=CARTESIAN_POINT('',(15.,8.26433068237712,14.7203487384281));
#77172=CARTESIAN_POINT('Origin',(15.,8.26786622031554,14.320364363769));
#77173=CARTESIAN_POINT('',(15.,3.93404948555832,14.6820725595938));
#77174=CARTESIAN_POINT('',(15.,8.5,14.7224318643355));
#77175=CARTESIAN_POINT('',(15.,0.203054053000302,16.8803613012335));
#77176=CARTESIAN_POINT('',(15.,3.93404948555832,14.6820725595938));
#77177=CARTESIAN_POINT('',(15.,-0.203054053000299,16.8803613012335));
#77178=CARTESIAN_POINT('Origin',(15.,8.32667268468867E-16,16.5357324406311));
#77179=CARTESIAN_POINT('',(15.,-3.93404948555832,14.6820725595938));
#77180=CARTESIAN_POINT('',(15.,1.04094977927525E-15,17.));
#77181=CARTESIAN_POINT('',(15.,-8.26433068237711,14.7203487384281));
#77182=CARTESIAN_POINT('',(15.,-3.93404948555832,14.6820725595938));
#77183=CARTESIAN_POINT('',(15.,-8.61603061885642,14.5172946854278));
#77184=CARTESIAN_POINT('Origin',(15.,-8.26786622031553,14.320364363769));
#77185=CARTESIAN_POINT('',(15.,-10.7480230740355,10.7480230740355));
#77186=CARTESIAN_POINT('',(15.,-8.5,14.7224318643355));
#77187=CARTESIAN_POINT('',(15.,-14.5172946854278,8.61603061885642));
#77188=CARTESIAN_POINT('',(15.,-10.7480230740355,10.7480230740355));
#77189=CARTESIAN_POINT('',(15.,-14.7203487384281,8.26433068237712));
#77190=CARTESIAN_POINT('Origin',(15.,-14.320364363769,8.26786622031554));
#77191=CARTESIAN_POINT('',(15.,-14.6820725595938,3.93404948555832));
#77192=CARTESIAN_POINT('',(15.,-14.7224318643355,8.5));
#77193=CARTESIAN_POINT('',(15.,-16.8803613012335,0.203054053000302));
#77194=CARTESIAN_POINT('',(15.,-14.6820725595938,3.93404948555832));
#77195=CARTESIAN_POINT('',(15.,-16.8803613012335,-0.203054053000298));
#77196=CARTESIAN_POINT('Origin',(15.,-16.5357324406311,2.22044604925031E-15));
#77197=CARTESIAN_POINT('',(15.,-14.6820725595938,-3.93404948555832));
#77198=CARTESIAN_POINT('',(15.,-17.,2.0818995585505E-15));
#77199=CARTESIAN_POINT('',(15.,-14.7203487384281,-8.26433068237712));
#77200=CARTESIAN_POINT('',(15.,-14.6820725595938,-3.93404948555832));
#77201=CARTESIAN_POINT('',(15.,-14.5172946854278,-8.61603061885642));
#77202=CARTESIAN_POINT('Origin',(15.,-14.320364363769,-8.26786622031554));
#77203=CARTESIAN_POINT('',(15.,-10.7480230740355,-10.7480230740355));
#77204=CARTESIAN_POINT('',(15.,-14.7224318643355,-8.5));
#77205=CARTESIAN_POINT('',(15.,-8.61603061885643,-14.5172946854278));
#77206=CARTESIAN_POINT('',(15.,-10.7480230740355,-10.7480230740355));
#77207=CARTESIAN_POINT('',(15.,-8.26433068237712,-14.7203487384281));
#77208=CARTESIAN_POINT('Origin',(15.,-8.26786622031554,-14.320364363769));
#77209=CARTESIAN_POINT('',(15.,-3.93404948555831,-14.6820725595938));
#77210=CARTESIAN_POINT('',(15.,-8.50000000000001,-14.7224318643355));
#77211=CARTESIAN_POINT('',(15.,-0.203054053000303,-16.8803613012335));
#77212=CARTESIAN_POINT('',(15.,-3.93404948555831,-14.6820725595938));
#77213=CARTESIAN_POINT('',(15.,0.203054053000297,-16.8803613012335));
#77214=CARTESIAN_POINT('Origin',(15.,-2.77555756156289E-15,-16.5357324406311));
#77215=CARTESIAN_POINT('',(15.,3.93404948555831,-14.6820725595938));
#77216=CARTESIAN_POINT('',(15.,-3.12284933782575E-15,-17.));
#77217=CARTESIAN_POINT('',(15.,8.26433068237712,-14.7203487384281));
#77218=CARTESIAN_POINT('',(15.,3.93404948555831,-14.6820725595938));
#77219=CARTESIAN_POINT('',(15.,8.61603061885642,-14.5172946854278));
#77220=CARTESIAN_POINT('Origin',(15.,8.26786622031554,-14.320364363769));
#77221=CARTESIAN_POINT('',(15.,10.7480230740355,-10.7480230740355));
#77222=CARTESIAN_POINT('',(15.,8.5,-14.7224318643355));
#77223=CARTESIAN_POINT('',(15.,14.5172946854278,-8.61603061885643));
#77224=CARTESIAN_POINT('',(15.,10.7480230740355,-10.7480230740355));
#77225=CARTESIAN_POINT('Origin',(15.,14.320364363769,-8.26786622031554));
#77226=CARTESIAN_POINT('Origin',(1.27397318515336,-8.26786622031553,14.320364363769));
#77227=CARTESIAN_POINT('',(1.27397318515336,-8.61603061885641,14.5172946854278));
#77228=CARTESIAN_POINT('',(1.27397318515336,-8.26433068237711,14.7203487384281));
#77229=CARTESIAN_POINT('Origin',(1.27397318515336,-8.26786622031553,14.320364363769));
#77230=CARTESIAN_POINT('',(0.975876659743318,-8.4012251922095,14.5513488787345));
#77231=CARTESIAN_POINT('Origin',(1.27397318515336,-8.26786622031553,14.320364363769));
#77232=CARTESIAN_POINT('Origin',(1.27397318515336,-8.26786622031553,14.320364363769));
#77233=CARTESIAN_POINT('Origin',(0.,-8.26786622031553,14.320364363769));
#77234=CARTESIAN_POINT('',(0.,-8.61603061885642,14.5172946854278));
#77235=CARTESIAN_POINT('',(0.,-8.26433068237711,14.7203487384281));
#77236=CARTESIAN_POINT('Origin',(0.,-8.5,14.7224318643355));
#77237=CARTESIAN_POINT('',(1.54223855908242E-12,-10.2674425839711,11.5976688566876));
#77238=CARTESIAN_POINT('Ctrl Pts',(1.73472347597681E-17,-10.2674425839761,
11.5976688566786));
#77239=CARTESIAN_POINT('Ctrl Pts',(0.342255094986008,-9.70275089163238,
12.596019652888));
#77240=CARTESIAN_POINT('Ctrl Pts',(0.778977013899441,-9.15257721870111,
13.568703210786));
#77241=CARTESIAN_POINT('Ctrl Pts',(1.27397318515336,-8.61603061885642,14.5172946854278));
#77242=CARTESIAN_POINT('',(0.,-11.1302408997889,10.0722782811866));
#77243=CARTESIAN_POINT('',(0.,-8.5,14.7224318643355));
#77244=CARTESIAN_POINT('',(0.4,-10.7480230740355,10.7480230740355));
#77245=CARTESIAN_POINT('Origin',(0.4,-11.1302408997889,10.0722782811866));
#77246=CARTESIAN_POINT('',(0.,-10.7480230740355,10.7480230740355));
#77247=CARTESIAN_POINT('Ctrl Pts',(0.975876659743318,-8.4012251922095,14.5513488787345));
#77248=CARTESIAN_POINT('Ctrl Pts',(0.480880488489402,-8.95088792863941,
13.5951847991044));
#77249=CARTESIAN_POINT('Ctrl Pts',(0.0441585695759696,-9.51525928157349,
12.6128343866363));
#77250=CARTESIAN_POINT('Ctrl Pts',(-0.29809652541004,-10.0943490218541,
11.6019564859438));
#77251=CARTESIAN_POINT('Ctrl Pts',(1.04274635983407,-8.50725783232391,14.5764294404348));
#77252=CARTESIAN_POINT('Ctrl Pts',(0.549500871257885,-9.05208409138169,
13.6199550988967));
#77253=CARTESIAN_POINT('Ctrl Pts',(0.114336878352,-9.61133007010324,12.6381777144107));
#77254=CARTESIAN_POINT('Ctrl Pts',(-0.2265329429665,-10.1852829938157,11.6288575090248));
#77255=CARTESIAN_POINT('Ctrl Pts',(1.15757519551698,-8.59000236282894,14.5633115305157));
#77256=CARTESIAN_POINT('Ctrl Pts',(0.663548261198223,-9.12920774203301,
13.6098465697466));
#77257=CARTESIAN_POINT('Ctrl Pts',(0.227656291976222,-9.68257776114536,
12.631808325544));
#77258=CARTESIAN_POINT('Ctrl Pts',(-0.113842189164374,-10.2507183220772,
11.6272366374857));
#77259=CARTESIAN_POINT('Ctrl Pts',(1.27397318515336,-8.61603061885642,14.5172946854278));
#77260=CARTESIAN_POINT('Ctrl Pts',(0.778977013899441,-9.15257721870111,
13.568703210786));
#77261=CARTESIAN_POINT('Ctrl Pts',(0.342255094986008,-9.70275089163238,
12.596019652888));
#77262=CARTESIAN_POINT('Ctrl Pts',(1.73472347597681E-17,-10.2674425839761,
11.5976688566786));
#77263=CARTESIAN_POINT('',(0.101903474589959,-9.48134128444654,12.6710528913746));
#77264=CARTESIAN_POINT('Ctrl Pts',(0.975876659743318,-8.4012251922095,14.5513488787345));
#77265=CARTESIAN_POINT('Ctrl Pts',(0.6571407874074,-8.75516173144116,13.9356596881592));
#77266=CARTESIAN_POINT('Ctrl Pts',(0.362567028519819,-9.11519686904806,
13.3091129212202));
#77267=CARTESIAN_POINT('Ctrl Pts',(0.101818266846041,-9.48133321370126,
12.6710835238972));
#77268=CARTESIAN_POINT('',(0.,-10.1523726680387,11.7902463207642));
#77269=CARTESIAN_POINT('Ctrl Pts',(0.10190347458996,-9.48134128444654,12.6710528913746));
#77270=CARTESIAN_POINT('Ctrl Pts',(0.101531854872349,-9.48275534163259,
12.6694760546067));
#77271=CARTESIAN_POINT('Ctrl Pts',(0.10116125464251,-9.48416877757454,12.6678984134383));
#77272=CARTESIAN_POINT('Ctrl Pts',(0.0322255740955127,-9.74769125598168,
12.3734824313406));
#77273=CARTESIAN_POINT('Ctrl Pts',(5.77268084014669E-16,-9.98134172659987,
12.0609347949683));
#77274=CARTESIAN_POINT('Ctrl Pts',(3.46944695195361E-17,-10.1523726680387,
11.7902463207642));
#77275=CARTESIAN_POINT('Ctrl Pts',(7.55756463219348E-5,-10.1522033136756,
11.7901117494112));
#77276=CARTESIAN_POINT('Ctrl Pts',(3.99782202685582E-5,-10.1883017538264,
11.7331721436165));
#77277=CARTESIAN_POINT('Ctrl Pts',(8.3791975840389E-6,-10.2229268058455,
11.6755689736335));
#77278=CARTESIAN_POINT('Ctrl Pts',(1.28003763560924E-6,-10.2559234055978,
11.6179147284068));
#77279=CARTESIAN_POINT('Ctrl Pts',(4.49108246820633E-7,-10.2597855307877,
11.6111665205772));
#77280=CARTESIAN_POINT('Ctrl Pts',(2.85831882484854E-12,-10.2636253415182,
11.6044175783242));
#77281=CARTESIAN_POINT('Ctrl Pts',(2.95841129371865E-12,-10.2674425839713,
11.5976688566872));
#77282=CARTESIAN_POINT('Ctrl Pts',(-0.29809652541004,-5.00041453950186,
14.5429409305642));
#77283=CARTESIAN_POINT('Ctrl Pts',(0.0441573423013372,-6.1654011742866,
14.546873440655));
#77284=CARTESIAN_POINT('Ctrl Pts',(0.48087971098951,-7.29832970851256,14.5492887289455));
#77285=CARTESIAN_POINT('Ctrl Pts',(0.975876659743318,-8.4012251922095,14.5513488787345));
#77286=CARTESIAN_POINT('Ctrl Pts',(-0.2265329429665,-4.97824452289702,14.6351425718904));
#77287=CARTESIAN_POINT('Ctrl Pts',(0.114335656044747,-6.13931375973807,
14.6427448348114));
#77288=CARTESIAN_POINT('Ctrl Pts',(0.549500096507824,-7.26918333939724,
14.6493123197193));
#77289=CARTESIAN_POINT('Ctrl Pts',(1.04274635983407,-8.36992927572593,14.655716119554));
#77290=CARTESIAN_POINT('Ctrl Pts',(-0.113842189164374,-4.94412314283721,
14.6910007927003));
#77291=CARTESIAN_POINT('Ctrl Pts',(0.227655067414694,-6.09817388681918,
14.7012624412453));
#77292=CARTESIAN_POINT('Ctrl Pts',(0.66354748522073,-7.2218672795407,14.7110490905584));
#77293=CARTESIAN_POINT('Ctrl Pts',(1.15757519551698,-8.31719656723893,14.7208160300361));
#77294=CARTESIAN_POINT('Ctrl Pts',(3.46944695195361E-17,-4.91015456257522,
14.6907005379608));
#77295=CARTESIAN_POINT('Ctrl Pts',(0.342253867711377,-6.05709344738998,
14.7008385488363));
#77296=CARTESIAN_POINT('Ctrl Pts',(0.778976236399549,-7.17455135586717,
14.7107159717565));
#77297=CARTESIAN_POINT('Ctrl Pts',(1.27397318515336,-8.26433068237711,14.7203487384281));
#77298=CARTESIAN_POINT('',(1.11810734282347E-12,-4.91015456258271,14.6907005379609));
#77299=CARTESIAN_POINT('Ctrl Pts',(1.27397318515336,-8.26433068237711,14.7203487384281));
#77300=CARTESIAN_POINT('Ctrl Pts',(0.778976236399549,-7.17455135586717,
14.7107159717565));
#77301=CARTESIAN_POINT('Ctrl Pts',(0.342253867711377,-6.05709344738998,
14.7008385488363));
#77302=CARTESIAN_POINT('Ctrl Pts',(3.46944695195361E-17,-4.91015456257522,
14.6907005379608));
#77303=CARTESIAN_POINT('',(0.,-5.13446649663842,14.6873357995904));
#77304=CARTESIAN_POINT('Ctrl Pts',(2.14489537242457E-12,-4.91015456258241,
14.6907005379609));
#77305=CARTESIAN_POINT('Ctrl Pts',(1.91519594125472E-12,-4.97672175417232,
14.691288938024));
#77306=CARTESIAN_POINT('Ctrl Pts',(3.02757473638156E-5,-5.04411570871069,
14.6904461671435));
#77307=CARTESIAN_POINT('Ctrl Pts',(6.40162742490125E-5,-5.11171923539963,
14.6880030229077));
#77308=CARTESIAN_POINT('Ctrl Pts',(6.77941797834191E-5,-5.11928875968396,
14.6877294655871));
#77309=CARTESIAN_POINT('Ctrl Pts',(7.16591806610037E-5,-5.12686088525319,
14.6874358249055));
#77310=CARTESIAN_POINT('Ctrl Pts',(7.56088218995532E-5,-5.13443472496738,
14.687121849529));
#77311=CARTESIAN_POINT('',(0.101903474589959,-6.23278305440342,14.5466088599682));
#77312=CARTESIAN_POINT('Ctrl Pts',(3.46944695195361E-17,-5.13446649663842,
14.6873357995904));
#77313=CARTESIAN_POINT('Ctrl Pts',(1.69204094774372E-17,-5.4544006361908,
14.674563073286));
#77314=CARTESIAN_POINT('Ctrl Pts',(0.0322246857018699,-5.84189399125915,
14.6284907480811));
#77315=CARTESIAN_POINT('Ctrl Pts',(0.101159446169479,-6.22862733387103,
14.5474824258378));
#77316=CARTESIAN_POINT('Ctrl Pts',(0.101530948145745,-6.23070538808735,
14.547046115306));
#77317=CARTESIAN_POINT('Ctrl Pts',(0.101903474589959,-6.23278305440342,
14.5466088599682));
#77318=CARTESIAN_POINT('Ctrl Pts',(0.101818330923698,-6.23281359529303,
14.546617185632));
#77319=CARTESIAN_POINT('Ctrl Pts',(0.362566764210783,-6.96843040513953,
14.5485485053788));
#77320=CARTESIAN_POINT('Ctrl Pts',(0.657140611963177,-7.69105405181532,
14.5500223170188));
#77321=CARTESIAN_POINT('Ctrl Pts',(0.975876659743318,-8.4012251922095,14.5513488787345));
#77322=CARTESIAN_POINT('Origin',(18.6,0.,0.));
#77323=CARTESIAN_POINT('',(19.,-2.1350877539664E-15,17.4343145750508));
#77324=CARTESIAN_POINT('Origin',(19.,0.,0.));
#77325=CARTESIAN_POINT('Origin',(18.6,-2.1350877539664E-15,17.4343145750508));
#77326=CARTESIAN_POINT('Origin',(19.,11.05,0.));
#77327=CARTESIAN_POINT('',(19.,-1.40222058502372E-15,11.45));
#77328=CARTESIAN_POINT('Origin',(19.,0.,0.));
#77329=CARTESIAN_POINT('Origin',(18.6,0.,0.));
#77330=CARTESIAN_POINT('',(18.6,-1.35323471305783E-15,11.05));
#77331=CARTESIAN_POINT('',(18.6,-11.05,-1.35323471305783E-15));
#77332=CARTESIAN_POINT('Origin',(18.6,0.,0.));
#77333=CARTESIAN_POINT('Origin',(18.6,0.,0.));
#77334=CARTESIAN_POINT('Origin',(18.6,-1.40222058502372E-15,11.45));
#77335=CARTESIAN_POINT('Origin',(17.,0.,0.));
#77336=CARTESIAN_POINT('',(0.978144961882947,-11.05,-1.35323471305783E-15));
#77337=CARTESIAN_POINT('',(17.,-11.05,-1.35323471305783E-15));
#77338=CARTESIAN_POINT('',(0.978144961882947,-1.35323471305783E-15,11.05));
#77339=CARTESIAN_POINT('Origin',(0.978144961882947,0.,0.));
#77340=CARTESIAN_POINT('Origin',(0.978144961882947,0.,0.));
#77341=CARTESIAN_POINT('Origin',(0.978144961882947,0.,0.));
#77342=CARTESIAN_POINT('',(0.680827303384081,-1.36945076433076E-15,11.182414107351));
#77343=CARTESIAN_POINT('',(0.680827303384083,-11.182414107351,-1.36945076433076E-15));
#77344=CARTESIAN_POINT('Origin',(0.680827303384081,0.,-1.71181345541345E-15));
#77345=CARTESIAN_POINT('Origin',(0.680827303384081,0.,-1.71181345541345E-15));
#77346=CARTESIAN_POINT('Origin',(0.978144961882947,-1.40222058502372E-15,
11.45));
#77347=CARTESIAN_POINT('Origin',(0.349999999999999,0.,0.));
#77348=CARTESIAN_POINT('',(0.102682341501134,-11.8247973983321,-2.89624005688666E-15));
#77349=CARTESIAN_POINT('',(0.102682341501134,-1.44812002844333E-15,11.8247973983321));
#77350=CARTESIAN_POINT('Origin',(0.102682341501134,0.,-7.24060014221666E-16));
#77351=CARTESIAN_POINT('',(0.349999999999999,-11.55,-1.41446705301519E-15));
#77352=CARTESIAN_POINT('Origin',(0.102682341501134,0.,-7.24060014221666E-16));
#77353=CARTESIAN_POINT('Origin',(0.,-14.320364363769,8.26786622031554));
#77354=CARTESIAN_POINT('',(1.27397318515336,-14.5172946854278,8.61603061885642));
#77355=CARTESIAN_POINT('',(1.27397318515336,-14.7203487384281,8.26433068237711));
#77356=CARTESIAN_POINT('Origin',(1.27397318515336,-14.320364363769,8.26786622031554));
#77357=CARTESIAN_POINT('',(0.,-14.7203487384281,8.26433068237712));
#77358=CARTESIAN_POINT('',(0.,-14.5172946854278,8.61603061885642));
#77359=CARTESIAN_POINT('Ctrl Pts',(0.101903474592389,-12.6710528913806,
9.48134128444314));
#77360=CARTESIAN_POINT('Ctrl Pts',(0.362758547479537,-13.3092044981173,
9.11512949353394));
#77361=CARTESIAN_POINT('Ctrl Pts',(0.65711604755494,-13.9356118991871,8.75518920352235));
#77362=CARTESIAN_POINT('Ctrl Pts',(0.975876659743319,-14.5513488787345,
8.4012251922095));
#77363=CARTESIAN_POINT('Ctrl Pts',(0.171922236292925,-12.6966530089968,
9.57774919679077));
#77364=CARTESIAN_POINT('Ctrl Pts',(0.431766345557849,-13.3343020570724,
9.21485636586833));
#77365=CARTESIAN_POINT('Ctrl Pts',(0.725113127440746,-13.9604926628253,
8.85810731755049));
#77366=CARTESIAN_POINT('Ctrl Pts',(1.04274635983407,-14.5764294404348,8.50725783232391));
#77367=CARTESIAN_POINT('Ctrl Pts',(0.285320162667741,-12.6903300945564,
9.6494065931016));
#77368=CARTESIAN_POINT('Ctrl Pts',(0.545620573531755,-13.3253566536154,
9.29027284840102));
#77369=CARTESIAN_POINT('Ctrl Pts',(0.839438738780195,-13.9493126912418,
8.93723219358695));
#77370=CARTESIAN_POINT('Ctrl Pts',(1.15757519551698,-14.5633115305157,8.59000236282894));
#77371=CARTESIAN_POINT('Ctrl Pts',(0.400000000002429,-12.6544314337809,
9.66971175595938));
#77372=CARTESIAN_POINT('Ctrl Pts',(0.660855072889578,-13.2857620430748,
9.31261568156927));
#77373=CARTESIAN_POINT('Ctrl Pts',(0.955212572964979,-13.9064342046133,
8.96154828660087));
#77374=CARTESIAN_POINT('Ctrl Pts',(1.27397318515336,-14.5172946854278,8.61603061885642));
#77375=CARTESIAN_POINT('',(0.975876659743319,-14.5513488787345,8.4012251922095));
#77376=CARTESIAN_POINT('Origin',(1.27397318515336,-14.320364363769,8.26786622031553));
#77377=CARTESIAN_POINT('',(0.400000000002429,-12.6544314337809,9.66971175595937));
#77378=CARTESIAN_POINT('Ctrl Pts',(1.27397318515336,-14.5172946854278,8.61603061885642));
#77379=CARTESIAN_POINT('Ctrl Pts',(0.955212572964979,-13.9064342046133,
8.96154828660087));
#77380=CARTESIAN_POINT('Ctrl Pts',(0.660855072889578,-13.2857620430748,
9.31261568156927));
#77381=CARTESIAN_POINT('Ctrl Pts',(0.400000000002429,-12.6544314337809,
9.66971175595938));
#77382=CARTESIAN_POINT('',(0.10190347459239,-12.6710528913795,9.48134128444232));
#77383=CARTESIAN_POINT('Origin',(0.400000000002429,-12.457501112122,9.32154735741849));
#77384=CARTESIAN_POINT('Ctrl Pts',(0.101903474592389,-12.6710528913806,
9.48134128444314));
#77385=CARTESIAN_POINT('Ctrl Pts',(0.362758547479537,-13.3092044981173,
9.11512949353394));
#77386=CARTESIAN_POINT('Ctrl Pts',(0.65711604755494,-13.9356118991871,8.75518920352235));
#77387=CARTESIAN_POINT('Ctrl Pts',(0.975876659743319,-14.5513488787345,
8.4012251922095));
#77388=CARTESIAN_POINT('Origin',(0.4,-8.78256193508806,11.4001830744621));
#77389=CARTESIAN_POINT('',(0.,-12.4575011121161,9.32154735742181));
#77390=CARTESIAN_POINT('Origin',(0.4,-12.4575011121161,9.32154735742182));
#77391=CARTESIAN_POINT('',(0.4,-8.97949225674692,11.748347473003));
#77392=CARTESIAN_POINT('',(0.,-8.78256193508806,11.4001830744621));
#77393=CARTESIAN_POINT('Origin',(0.4,-12.4575011121161,9.32154735742182));
#77394=CARTESIAN_POINT('Origin',(0.4,-12.4575011121161,9.32154735742182));
#77395=CARTESIAN_POINT('Origin',(1.27397318515336,-14.320364363769,8.26786622031554));
#77396=CARTESIAN_POINT('Origin',(1.27397318515336,-14.320364363769,8.26786622031554));
#77397=CARTESIAN_POINT('Origin',(0.,-14.7224318643355,8.5));
#77398=CARTESIAN_POINT('',(0.400000000002955,-14.7014317448244,6.12420321413256));
#77399=CARTESIAN_POINT('Ctrl Pts',(0.400000000000004,-14.7014317448242,
6.12420321411614));
#77400=CARTESIAN_POINT('Ctrl Pts',(0.660836697158376,-14.7078423258376,
6.84944850421848));
#77401=CARTESIAN_POINT('Ctrl Pts',(0.95520620877991,-14.7141454518953,7.56253714263826));
#77402=CARTESIAN_POINT('Ctrl Pts',(1.27397318515336,-14.7203487384281,8.26433068237712));
#77403=CARTESIAN_POINT('',(0.4,-14.6820725595938,3.93404948555832));
#77404=CARTESIAN_POINT('',(0.4,-14.6842931448515,4.18526992814785));
#77405=CARTESIAN_POINT('',(0.,-14.6820725595938,3.93404948555832));
#77406=CARTESIAN_POINT('Ctrl Pts',(0.97587665974332,-14.5513488787345,8.4012251922095));
#77407=CARTESIAN_POINT('Ctrl Pts',(0.657109683369871,-14.5500221882957,
7.69098514026757));
#77408=CARTESIAN_POINT('Ctrl Pts',(0.362740171748336,-14.5485358134915,
6.96849262263025));
#77409=CARTESIAN_POINT('Ctrl Pts',(0.101903474589965,-14.5466088599682,
6.23278305440344));
#77410=CARTESIAN_POINT('Ctrl Pts',(1.04274635983407,-14.655716119554,8.36992927572593));
#77411=CARTESIAN_POINT('Ctrl Pts',(0.725106785764273,-14.6515922155264,
7.66107348426656));
#77412=CARTESIAN_POINT('Ctrl Pts',(0.431748041043186,-14.6474504130738,
6.94036445765127));
#77413=CARTESIAN_POINT('Ctrl Pts',(0.17192223629051,-14.6429006199952,6.20674945042513));
#77414=CARTESIAN_POINT('Ctrl Pts',(1.15757519551698,-14.7208160300361,8.31719656723893));
#77415=CARTESIAN_POINT('Ctrl Pts',(0.839432387056643,-14.7145263392136,
7.61182897648535));
#77416=CARTESIAN_POINT('Ctrl Pts',(0.545602236873285,-14.7082901641236,
6.89490956213576));
#77417=CARTESIAN_POINT('Ctrl Pts',(0.285320162665322,-14.7017962883492,
6.16544494773845));
#77418=CARTESIAN_POINT('Ctrl Pts',(1.27397318515336,-14.7203487384281,8.26433068237712));
#77419=CARTESIAN_POINT('Ctrl Pts',(0.95520620877991,-14.7141454518953,7.56253714263826));
#77420=CARTESIAN_POINT('Ctrl Pts',(0.660836697158376,-14.7078423258376,
6.84944850421848));
#77421=CARTESIAN_POINT('Ctrl Pts',(0.400000000000004,-14.7014317448242,
6.12420321411614));
#77422=CARTESIAN_POINT('',(0.101903474589965,-14.5466088599682,6.23278305440343));
#77423=CARTESIAN_POINT('Ctrl Pts',(0.97587665974332,-14.5513488787345,8.4012251922095));
#77424=CARTESIAN_POINT('Ctrl Pts',(0.657109683369871,-14.5500221882957,
7.69098514026757));
#77425=CARTESIAN_POINT('Ctrl Pts',(0.362740171748336,-14.5485358134915,
6.96849262263025));
#77426=CARTESIAN_POINT('Ctrl Pts',(0.101903474589965,-14.5466088599682,
6.23278305440344));
#77427=CARTESIAN_POINT('Origin',(0.400000000005235,-14.3014473701652,6.1277387520691));
#77428=CARTESIAN_POINT('Origin',(0.75,0.,0.));
#77429=CARTESIAN_POINT('Origin',(0.101903474589961,0.,0.));
#77430=CARTESIAN_POINT('Origin',(0.4,0.,0.));
#77431=CARTESIAN_POINT('',(0.,-14.3014473701651,6.12773875205456));
#77432=CARTESIAN_POINT('Origin',(0.,0.,0.));
#77433=CARTESIAN_POINT('Origin',(0.4,-14.3014473701651,6.12773875205456));
#77434=CARTESIAN_POINT('Origin',(0.,0.,0.));
#77435=CARTESIAN_POINT('Origin',(0.,0.,0.));
#77436=CARTESIAN_POINT('',(0.,-3.1577284155994,14.6752105100511));
#77437=CARTESIAN_POINT('',(0.,-3.93404948555832,14.6820725595938));
#77438=CARTESIAN_POINT('',(0.,-1.84394625804893,15.4492861094764));
#77439=CARTESIAN_POINT('',(0.,-3.51454243995435,14.4649770035306));
#77440=CARTESIAN_POINT('',(0.,1.84394625803322,15.4492861094856));
#77441=CARTESIAN_POINT('Origin',(0.,0.,0.));
#77442=CARTESIAN_POINT('',(0.,3.82661115890557,14.2811072658456));
#77443=CARTESIAN_POINT('',(0.,5.48156718273351,13.3060132833275));
#77444=CARTESIAN_POINT('',(0.,6.12773875205455,14.3014473701651));
#77445=CARTESIAN_POINT('',(0.,4.18880546608628,14.2843087701924));
#77446=CARTESIAN_POINT('',(0.,9.32154735741501,12.4575011121282));
#77447=CARTESIAN_POINT('Origin',(0.,0.,0.));
#77448=CARTESIAN_POINT('',(0.,10.0722782811866,11.1302408997889));
#77449=CARTESIAN_POINT('',(0.,11.4001830744621,8.78256193508806));
#77450=CARTESIAN_POINT('',(1.5421171284391E-12,11.5976688566876,10.2674425839711));
#77451=CARTESIAN_POINT('',(0.,14.7224318643355,8.5));
#77452=CARTESIAN_POINT('',(0.,11.7902463207642,10.1523726680387));
#77453=CARTESIAN_POINT('Ctrl Pts',(7.55756463215462E-5,11.7901117494112,
10.1522033136756));
#77454=CARTESIAN_POINT('Ctrl Pts',(3.99782202683874E-5,11.7331721436165,
10.1883017538264));
#77455=CARTESIAN_POINT('Ctrl Pts',(8.37919758296273E-6,11.6755689736335,
10.2229268058455));
#77456=CARTESIAN_POINT('Ctrl Pts',(1.28003763549822E-6,11.6179147284067,
10.2559234055978));
#77457=CARTESIAN_POINT('Ctrl Pts',(4.49108246825123E-7,11.6111665205772,
10.2597855307877));
#77458=CARTESIAN_POINT('Ctrl Pts',(2.85806772813845E-12,11.6044175783242,
10.2636253415182));
#77459=CARTESIAN_POINT('Ctrl Pts',(2.95818924911373E-12,11.5976688566872,
10.2674425839713));
#77460=CARTESIAN_POINT('',(0.,14.6873357995904,5.13446649663844));
#77461=CARTESIAN_POINT('Origin',(0.,0.,0.));
#77462=CARTESIAN_POINT('',(1.83636092443429E-12,14.6907005379609,4.91015456258753));
#77463=CARTESIAN_POINT('Ctrl Pts',(3.52262663483316E-12,14.6907005379609,
4.91015456258702));
#77464=CARTESIAN_POINT('Ctrl Pts',(3.14384478636717E-12,14.691289389039,
4.97677277863876));
#77465=CARTESIAN_POINT('Ctrl Pts',(3.0421313568722E-5,14.6904448446972,
5.04421606720833));
#77466=CARTESIAN_POINT('Ctrl Pts',(6.42665025712974E-5,14.6879977771591,
5.11186540275618));
#77467=CARTESIAN_POINT('Ctrl Pts',(6.80293897049442E-5,14.6877257137071,
5.11938661394851));
#77468=CARTESIAN_POINT('Ctrl Pts',(7.18776565831689E-5,14.6874338227259,
5.12691034625046));
#77469=CARTESIAN_POINT('Ctrl Pts',(7.58086218434206E-5,14.6871218582888,
5.13443572864623));
#77470=CARTESIAN_POINT('',(0.,14.6820725595938,3.93404948555832));
#77471=CARTESIAN_POINT('',(0.,14.6820725595938,3.93404948555832));
#77472=CARTESIAN_POINT('',(1.23108988281384E-12,15.1775971465556,3.09303168127507));
#77473=CARTESIAN_POINT('',(0.,17.,0.));
#77474=CARTESIAN_POINT('',(0.,15.2868391646771,2.89708947882623));
#77475=CARTESIAN_POINT('Ctrl Pts',(7.56025598233623E-5,15.2866379835645,
2.89701003430714));
#77476=CARTESIAN_POINT('Ctrl Pts',(3.99935540440351E-5,15.2553748760369,
2.95674426005502));
#77477=CARTESIAN_POINT('Ctrl Pts',(8.37940696159955E-6,15.2228002172963,
3.01553438614584));
#77478=CARTESIAN_POINT('Ctrl Pts',(1.27963547774668E-6,15.1893669609634,
3.07293977358698));
#77479=CARTESIAN_POINT('Ctrl Pts',(4.48956353211719E-7,15.185455242373,
3.07965625130625));
#77480=CARTESIAN_POINT('Ctrl Pts',(2.28183272822237E-12,15.1815317377524,
3.08635378609856));
#77481=CARTESIAN_POINT('Ctrl Pts',(2.36172192913386E-12,15.1775971465554,
3.09303168127536));
#77482=CARTESIAN_POINT('',(0.,15.2868391646771,-2.89708947882622));
#77483=CARTESIAN_POINT('Origin',(0.,0.,0.));
#77484=CARTESIAN_POINT('',(1.23111590366598E-12,15.1775971465556,-3.09303168127508));
#77485=CARTESIAN_POINT('Ctrl Pts',(2.36133335107525E-12,15.1775971465554,
-3.09303168127537));
#77486=CARTESIAN_POINT('Ctrl Pts',(2.1076010327172E-12,15.2114119674635,
-3.03564024767013));
#77487=CARTESIAN_POINT('Ctrl Pts',(3.03584523259135E-5,15.2443982679497,
-2.97681778667571));
#77488=CARTESIAN_POINT('Ctrl Pts',(6.40873890769833E-5,15.2761002062528,
-2.91701558164976));
#77489=CARTESIAN_POINT('Ctrl Pts',(6.7841766797752E-5,15.2796289581892,
-2.9103589808841));
#77490=CARTESIAN_POINT('Ctrl Pts',(7.16810510145227E-5,15.2831417674917,
-2.903690254015));
#77491=CARTESIAN_POINT('Ctrl Pts',(7.56025598233345E-5,15.2866379835645,
-2.89701003430714));
#77492=CARTESIAN_POINT('',(0.,14.2879693153883,-4.60293222886448));
#77493=CARTESIAN_POINT('',(0.,14.6820725595938,-3.93404948555831));
#77494=CARTESIAN_POINT('',(0.,14.3014473701651,-6.12773875205455));
#77495=CARTESIAN_POINT('',(0.,14.2843087701924,-4.18880546608629));
#77496=CARTESIAN_POINT('',(0.,12.4575011121161,-9.32154735742182));
#77497=CARTESIAN_POINT('Origin',(0.,0.,0.));
#77498=CARTESIAN_POINT('',(0.,10.45449610694,-10.45449610694));
#77499=CARTESIAN_POINT('',(0.,8.78256193508805,-11.4001830744621));
#77500=CARTESIAN_POINT('',(0.,9.32154735742182,-12.4575011121161));
#77501=CARTESIAN_POINT('',(0.,10.2761715374443,-10.769766330238));
#77502=CARTESIAN_POINT('',(0.,6.12773875205454,-14.3014473701651));
#77503=CARTESIAN_POINT('Origin',(0.,0.,0.));
#77504=CARTESIAN_POINT('',(0.,3.82661115890556,-14.2811072658456));
#77505=CARTESIAN_POINT('',(0.,1.90583020886544,-14.2641291178216));
#77506=CARTESIAN_POINT('',(0.,1.84394625804894,-15.4492861094764));
#77507=CARTESIAN_POINT('',(0.,3.51454243995435,-14.4649770035306));
#77508=CARTESIAN_POINT('',(0.,-1.84394625804895,-15.4492861094764));
#77509=CARTESIAN_POINT('Origin',(0.,0.,0.));
#77510=CARTESIAN_POINT('',(0.,-3.82661115890556,-14.2811072658456));
#77511=CARTESIAN_POINT('',(0.,-5.48156718273351,-13.3060132833275));
#77512=CARTESIAN_POINT('',(0.,-6.12773875205454,-14.3014473701651));
#77513=CARTESIAN_POINT('',(0.,-4.18880546608629,-14.2843087701924));
#77514=CARTESIAN_POINT('',(0.,-9.32154735742183,-12.4575011121161));
#77515=CARTESIAN_POINT('Origin',(0.,0.,0.));
#77516=CARTESIAN_POINT('',(0.,-10.45449610694,-10.45449610694));
#77517=CARTESIAN_POINT('',(0.,-11.4001830744621,-8.78256193508805));
#77518=CARTESIAN_POINT('',(0.,-12.4575011121161,-9.32154735742182));
#77519=CARTESIAN_POINT('',(0.,-10.769766330238,-10.2761715374443));
#77520=CARTESIAN_POINT('',(0.,-14.3014473701651,-6.12773875205454));
#77521=CARTESIAN_POINT('Origin',(0.,0.,0.));
#77522=CARTESIAN_POINT('',(0.,-14.2811072658456,-3.82661115890556));
#77523=CARTESIAN_POINT('',(0.,-14.2641291178216,-1.90583020886544));
#77524=CARTESIAN_POINT('',(0.,-15.4492861094764,-1.84394625804894));
#77525=CARTESIAN_POINT('',(0.,-14.4649770035306,-3.51454243995435));
#77526=CARTESIAN_POINT('',(0.,-15.4492861094764,1.84394625804894));
#77527=CARTESIAN_POINT('Origin',(0.,0.,0.));
#77528=CARTESIAN_POINT('',(0.,-14.2811072658456,3.82661115890556));
#77529=CARTESIAN_POINT('',(0.,-13.3060132833275,5.48156718273351));
#77530=CARTESIAN_POINT('',(0.,-14.2843087701924,4.18880546608627));
#77531=CARTESIAN_POINT('',(0.,-1.48088984913629E-15,12.0923832909811));
#77532=CARTESIAN_POINT('Origin',(0.,0.,0.));
#77533=CARTESIAN_POINT('Origin',(0.4,-15.4492861094764,1.84394625804894));
#77534=CARTESIAN_POINT('',(0.10190347458996,-15.71412433885,1.87555596859357));
#77535=CARTESIAN_POINT('',(0.4,-15.7939149700788,2.04700031104924));
#77536=CARTESIAN_POINT('Origin',(0.4,-15.4492861094764,1.84394625804894));
#77537=CARTESIAN_POINT('Origin',(0.4,-15.4492861094764,1.84394625804894));
#77538=CARTESIAN_POINT('Origin',(0.4,-15.4492861094764,1.84394625804894));
#77539=CARTESIAN_POINT('Ctrl Pts',(0.101903474596431,-15.7141243388591,
1.87555596857779));
#77540=CARTESIAN_POINT('Ctrl Pts',(0.362758547482579,-16.0836739463024,
1.23933145112007));
#77541=CARTESIAN_POINT('Ctrl Pts',(0.657116047556583,-16.4461885237397,
0.614410315592906));
#77542=CARTESIAN_POINT('Ctrl Pts',(0.975876659743315,-16.802450384419,5.41233724504764E-15));
#77543=CARTESIAN_POINT('Ctrl Pts',(0.171922236296951,-15.7844986472285,
1.94624761098862));
#77544=CARTESIAN_POINT('Ctrl Pts',(0.431766345560878,-16.1552725060978,
1.31314867652409));
#77545=CARTESIAN_POINT('Ctrl Pts',(0.725113127442384,-16.5191949541301,
0.691099635031739));
#77546=CARTESIAN_POINT('Ctrl Pts',(1.04274635983406,-16.8771871080498,0.0792866791192721));
#77547=CARTESIAN_POINT('Ctrl Pts',(0.285320162671774,-15.8148515408526,
2.01146619378309));
#77548=CARTESIAN_POINT('Ctrl Pts',(0.54562057353479,-16.1852338007232,1.38293396799004));
#77549=CARTESIAN_POINT('Ctrl Pts',(0.839438738781837,-16.5490752527434,
0.765213773542398));
#77550=CARTESIAN_POINT('Ctrl Pts',(1.15757519551697,-16.9071989300679,0.157504499520391));
#77551=CARTESIAN_POINT('Ctrl Pts',(0.400000000006471,-15.793914970088,2.04700031103374));
#77552=CARTESIAN_POINT('Ctrl Pts',(0.660855072892618,-16.1621152787262,
1.42208073437658));
#77553=CARTESIAN_POINT('Ctrl Pts',(0.955212572966624,-16.5240994405542,
0.807711371127489));
#77554=CARTESIAN_POINT('Ctrl Pts',(1.27397318515335,-16.8803613012335,0.203054053000305));
#77555=CARTESIAN_POINT('',(0.975876659743315,-16.802450384419,5.41233724504764E-15));
#77556=CARTESIAN_POINT('',(1.27397318515335,-16.8803613012335,0.203054053000303));
#77557=CARTESIAN_POINT('Origin',(1.27397318515335,-16.5357324406311,5.55111512312578E-15));
#77558=CARTESIAN_POINT('Ctrl Pts',(1.27397318515335,-16.8803613012335,0.203054053000305));
#77559=CARTESIAN_POINT('Ctrl Pts',(0.955212572966624,-16.5240994405542,
0.807711371127489));
#77560=CARTESIAN_POINT('Ctrl Pts',(0.660855072892618,-16.1621152787262,
1.42208073437658));
#77561=CARTESIAN_POINT('Ctrl Pts',(0.400000000006471,-15.793914970088,2.04700031103374));
#77562=CARTESIAN_POINT('Ctrl Pts',(0.101903474596431,-15.7141243388591,
1.87555596857779));
#77563=CARTESIAN_POINT('Ctrl Pts',(0.362758547482579,-16.0836739463024,
1.23933145112007));
#77564=CARTESIAN_POINT('Ctrl Pts',(0.657116047556583,-16.4461885237397,
0.614410315592906));
#77565=CARTESIAN_POINT('Ctrl Pts',(0.975876659743315,-16.802450384419,5.41233724504764E-15));
#77566=CARTESIAN_POINT('Origin',(0.4,-14.4649770035306,-3.51454243995435));
#77567=CARTESIAN_POINT('',(0.4,-15.7939149700788,-2.04700031104924));
#77568=CARTESIAN_POINT('Origin',(0.4,-15.4492861094764,-1.84394625804894));
#77569=CARTESIAN_POINT('',(0.4,-14.6820725595938,-3.93404948555832));
#77570=CARTESIAN_POINT('Origin',(0.4,-14.2811072658456,-3.82661115890556));
#77571=CARTESIAN_POINT('',(0.4,-14.8096058641331,-3.71759649295465));
#77572=CARTESIAN_POINT('Ctrl Pts',(0.975876659743317,-16.802450384419,2.4980018054066E-15));
#77573=CARTESIAN_POINT('Ctrl Pts',(0.657116047554946,-16.4461885237379,
-0.614410315596059));
#77574=CARTESIAN_POINT('Ctrl Pts',(0.362758547479549,-16.0836739462987,
-1.2393314511265));
#77575=CARTESIAN_POINT('Ctrl Pts',(0.101903474592405,-15.7141243388534,
-1.87555596858761));
#77576=CARTESIAN_POINT('Ctrl Pts',(1.04274635983407,-16.8771871080498,-0.0792866791192642));
#77577=CARTESIAN_POINT('Ctrl Pts',(0.725113127440752,-16.5191949541282,
-0.69109963503488));
#77578=CARTESIAN_POINT('Ctrl Pts',(0.431766345557859,-16.155272506094,-1.31314867653048));
#77579=CARTESIAN_POINT('Ctrl Pts',(0.17192223629294,-15.7844986472227,-1.94624761099839));
#77580=CARTESIAN_POINT('Ctrl Pts',(1.15757519551697,-16.9071989300679,-0.157504499520383));
#77581=CARTESIAN_POINT('Ctrl Pts',(0.839438738780201,-16.5490752527415,
-0.765213773545517));
#77582=CARTESIAN_POINT('Ctrl Pts',(0.545620573531767,-16.1852338007194,
-1.38293396799639));
#77583=CARTESIAN_POINT('Ctrl Pts',(0.285320162667756,-15.8148515408469,
-2.01146619379279));
#77584=CARTESIAN_POINT('Ctrl Pts',(1.27397318515336,-16.8803613012335,-0.203054053000297));
#77585=CARTESIAN_POINT('Ctrl Pts',(0.955212572964985,-16.5240994405524,
-0.807711371130593));
#77586=CARTESIAN_POINT('Ctrl Pts',(0.660855072889588,-16.1621152787225,
-1.42208073438289));
#77587=CARTESIAN_POINT('Ctrl Pts',(0.400000000002444,-15.7939149700823,
-2.04700031104338));
#77588=CARTESIAN_POINT('',(0.101903474592405,-15.7141243388521,-1.87555596858744));
#77589=CARTESIAN_POINT('Origin',(0.400000000002444,-15.4492861094798,-1.84394625804308));
#77590=CARTESIAN_POINT('',(1.27397318515336,-16.8803613012335,-0.203054053000298));
#77591=CARTESIAN_POINT('Ctrl Pts',(0.400000000002444,-15.7939149700823,
-2.04700031104338));
#77592=CARTESIAN_POINT('Ctrl Pts',(0.660855072889588,-16.1621152787225,
-1.42208073438289));
#77593=CARTESIAN_POINT('Ctrl Pts',(0.955212572964985,-16.5240994405524,
-0.807711371130593));
#77594=CARTESIAN_POINT('Ctrl Pts',(1.27397318515336,-16.8803613012335,-0.203054053000297));
#77595=CARTESIAN_POINT('Origin',(1.27397318515336,-16.5357324406311,2.08166817117217E-15));
#77596=CARTESIAN_POINT('Ctrl Pts',(0.975876659743317,-16.802450384419,2.4980018054066E-15));
#77597=CARTESIAN_POINT('Ctrl Pts',(0.657116047554946,-16.4461885237379,
-0.614410315596059));
#77598=CARTESIAN_POINT('Ctrl Pts',(0.362758547479549,-16.0836739462987,
-1.2393314511265));
#77599=CARTESIAN_POINT('Ctrl Pts',(0.101903474592405,-15.7141243388534,
-1.87555596858761));
#77600=CARTESIAN_POINT('Origin',(0.4,-15.4492861094771,-1.84394625804276));
#77601=CARTESIAN_POINT('Origin',(0.4,-15.4492861094771,-1.84394625804276));
#77602=CARTESIAN_POINT('Origin',(1.27397318515335,-16.5357324406311,2.22044604925031E-15));
#77603=CARTESIAN_POINT('Origin',(1.27397318515335,-16.5357324406311,2.22044604925031E-15));
#77604=CARTESIAN_POINT('Origin',(0.,-14.6820725595938,3.93404948555832));
#77605=CARTESIAN_POINT('',(0.,-16.8803613012335,0.203054053000302));
#77606=CARTESIAN_POINT('',(0.4,-13.65064214393,5.68462123573381));
#77607=CARTESIAN_POINT('Origin',(0.,-16.5357324406311,2.22044604925031E-15));
#77608=CARTESIAN_POINT('',(0.,-16.8803613012335,-0.203054053000297));
#77609=CARTESIAN_POINT('Origin',(0.,-17.,2.0818995585505E-15));
#77610=CARTESIAN_POINT('',(0.,-14.6820725595938,-3.93404948555832));
#77611=CARTESIAN_POINT('Origin',(0.4,14.2843087701924,-4.18880546608629));
#77612=CARTESIAN_POINT('',(0.4,14.7014317448242,-6.12420321411613));
#77613=CARTESIAN_POINT('Origin',(0.4,14.3014473701651,-6.12773875205455));
#77614=CARTESIAN_POINT('',(0.4,14.6820725595938,-3.93404948555831));
#77615=CARTESIAN_POINT('Origin',(0.4,14.2879693153883,-4.60293222886448));
#77616=CARTESIAN_POINT('',(0.4,14.6842931448515,-4.18526992814787));
#77617=CARTESIAN_POINT('Ctrl Pts',(0.975876659743318,14.5513488787345,-8.40122519220951));
#77618=CARTESIAN_POINT('Ctrl Pts',(0.657116047555016,14.5500222147831,-7.6909993202157));
#77619=CARTESIAN_POINT('Ctrl Pts',(0.362758547479679,14.5485359492438,-6.96854445276509));
#77620=CARTESIAN_POINT('Ctrl Pts',(0.101903474592579,14.5466088599682,-6.23278305441081));
#77621=CARTESIAN_POINT('Ctrl Pts',(1.04274635983407,14.655716119554,-8.36992927572594));
#77622=CARTESIAN_POINT('Ctrl Pts',(0.725113127440822,14.6515922978602,-7.66108763657792));
#77623=CARTESIAN_POINT('Ctrl Pts',(0.43176634555799,14.6474507336029,-6.94041614022602));
#77624=CARTESIAN_POINT('Ctrl Pts',(0.171922236293114,14.6429006199952,-6.20674945043248));
#77625=CARTESIAN_POINT('Ctrl Pts',(1.15757519551698,14.7208160300361,-8.31719656723894));
#77626=CARTESIAN_POINT('Ctrl Pts',(0.839438738780273,14.7145264647873,-7.61184305915476));
#77627=CARTESIAN_POINT('Ctrl Pts',(0.545620573531897,14.7082906216118,-6.89496095231874));
#77628=CARTESIAN_POINT('Ctrl Pts',(0.285320162667931,14.7017962883493,-6.16544494774577));
#77629=CARTESIAN_POINT('Ctrl Pts',(1.27397318515336,14.7203487384281,-8.26433068237712));
#77630=CARTESIAN_POINT('Ctrl Pts',(0.955212572965057,14.7141455757439,-7.56255115395171));
#77631=CARTESIAN_POINT('Ctrl Pts',(0.66085507288972,14.7078427774577,-6.84949959715354));
#77632=CARTESIAN_POINT('Ctrl Pts',(0.400000000002619,14.7014317448243,-6.12420321412341));
#77633=CARTESIAN_POINT('',(0.101903474592579,14.5466088599669,-6.23278305441024));
#77634=CARTESIAN_POINT('Origin',(0.400000000002619,14.3014473701651,-6.12773875206183));
#77635=CARTESIAN_POINT('',(1.27397318515336,14.7203487384281,-8.26433068237712));
#77636=CARTESIAN_POINT('Ctrl Pts',(0.400000000002619,14.7014317448243,-6.12420321412341));
#77637=CARTESIAN_POINT('Ctrl Pts',(0.66085507288972,14.7078427774577,-6.84949959715354));
#77638=CARTESIAN_POINT('Ctrl Pts',(0.955212572965057,14.7141455757439,-7.56255115395171));
#77639=CARTESIAN_POINT('Ctrl Pts',(1.27397318515336,14.7203487384281,-8.26433068237712));
#77640=CARTESIAN_POINT('',(0.975876659743316,14.5513488787345,-8.40122519220951));
#77641=CARTESIAN_POINT('Origin',(1.27397318515336,14.320364363769,-8.26786622031554));
#77642=CARTESIAN_POINT('Ctrl Pts',(0.975876659743318,14.5513488787345,-8.40122519220951));
#77643=CARTESIAN_POINT('Ctrl Pts',(0.657116047555016,14.5500222147831,-7.6909993202157));
#77644=CARTESIAN_POINT('Ctrl Pts',(0.362758547479679,14.5485359492438,-6.96854445276509));
#77645=CARTESIAN_POINT('Ctrl Pts',(0.101903474592579,14.5466088599682,-6.23278305441081));
#77646=CARTESIAN_POINT('Origin',(0.4,14.3014473701624,-6.12773875206068));
#77647=CARTESIAN_POINT('Origin',(0.4,14.3014473701624,-6.12773875206068));
#77648=CARTESIAN_POINT('Origin',(0.,14.320364363769,-8.26786622031554));
#77649=CARTESIAN_POINT('',(1.27397318515336,14.5172946854278,-8.61603061885642));
#77650=CARTESIAN_POINT('Origin',(1.27397318515336,14.320364363769,-8.26786622031554));
#77651=CARTESIAN_POINT('',(0.,14.7203487384281,-8.26433068237712));
#77652=CARTESIAN_POINT('',(0.,14.5172946854278,-8.61603061885643));
#77653=CARTESIAN_POINT('Origin',(1.27397318515336,14.320364363769,-8.26786622031554));
#77654=CARTESIAN_POINT('Origin',(1.27397318515336,14.320364363769,-8.26786622031554));
#77655=CARTESIAN_POINT('Origin',(0.4,0.,0.));
#77656=CARTESIAN_POINT('',(0.101903474593112,12.6710528913809,-9.48134128444107));
#77657=CARTESIAN_POINT('Origin',(0.10190347458996,0.,5.55111512312578E-16));
#77658=CARTESIAN_POINT('Origin',(0.4,12.4575011121161,-9.32154735742182));
#77659=CARTESIAN_POINT('Origin',(0.75,0.,0.));
#77660=CARTESIAN_POINT('Ctrl Pts',(0.101903474593111,12.6710528913823,-9.48134128444213));
#77661=CARTESIAN_POINT('Ctrl Pts',(0.362758167198481,13.3092035678037,-9.11513002740676));
#77662=CARTESIAN_POINT('Ctrl Pts',(0.657121637769337,13.9356226975781,-8.75518299593385));
#77663=CARTESIAN_POINT('Ctrl Pts',(0.975876659743322,14.5513488787345,-8.4012251922095));
#77664=CARTESIAN_POINT('Ctrl Pts',(0.101903474593111,12.6710528913823,-9.48134128444213));
#77665=CARTESIAN_POINT('Ctrl Pts',(0.362758167198481,13.3092035678037,-9.11513002740676));
#77666=CARTESIAN_POINT('Ctrl Pts',(0.657121637769337,13.9356226975781,-8.75518299593385));
#77667=CARTESIAN_POINT('Ctrl Pts',(0.975876659743322,14.5513488787345,-8.4012251922095));
#77668=CARTESIAN_POINT('Ctrl Pts',(0.171922236293644,12.6966530089985,-9.57774919678977));
#77669=CARTESIAN_POINT('Ctrl Pts',(0.4317659667506,13.3343011274915,-9.21485689490269));
#77670=CARTESIAN_POINT('Ctrl Pts',(0.725118697883897,13.9605034647202,-8.8581011645825));
#77671=CARTESIAN_POINT('Ctrl Pts',(1.04274635983407,14.5764294404348,-8.50725783232391));
#77672=CARTESIAN_POINT('Ctrl Pts',(0.285320162668462,12.6903300945582,-9.64940659310061));
#77673=CARTESIAN_POINT('Ctrl Pts',(0.545620194059298,13.3253557278576,-9.29027337195529));
#77674=CARTESIAN_POINT('Ctrl Pts',(0.839444318048564,13.9493234591504,-8.93722610409809));
#77675=CARTESIAN_POINT('Ctrl Pts',(1.15757519551698,14.5633115305157,-8.59000236282895));
#77676=CARTESIAN_POINT('Ctrl Pts',(0.400000000003151,12.6544314337826,-9.66971175595839));
#77677=CARTESIAN_POINT('Ctrl Pts',(0.66085469260852,13.285761122705,-9.31261620215297));
#77678=CARTESIAN_POINT('Ctrl Pts',(0.955218163179377,13.9064449174835,-8.9615422271388));
#77679=CARTESIAN_POINT('Ctrl Pts',(1.27397318515336,14.5172946854278,-8.61603061885642));
#77680=CARTESIAN_POINT('',(0.400000000003151,12.6544314337826,-9.66971175595839));
#77681=CARTESIAN_POINT('Ctrl Pts',(1.27397318515336,14.5172946854278,-8.61603061885642));
#77682=CARTESIAN_POINT('Ctrl Pts',(0.955218163179377,13.9064449174835,-8.9615422271388));
#77683=CARTESIAN_POINT('Ctrl Pts',(0.66085469260852,13.285761122705,-9.31261620215297));
#77684=CARTESIAN_POINT('Ctrl Pts',(0.400000000003151,12.6544314337826,-9.66971175595839));
#77685=CARTESIAN_POINT('Origin',(0.400000000003151,12.4575011121237,-9.32154735741751));
#77686=CARTESIAN_POINT('Origin',(0.,10.7480230740355,-10.7480230740355));
#77687=CARTESIAN_POINT('',(0.4,10.7480230740355,-10.7480230740355));
#77688=CARTESIAN_POINT('',(0.,10.7480230740355,-10.7480230740355));
#77689=CARTESIAN_POINT('',(0.4,8.97949225674692,-11.748347473003));
#77690=CARTESIAN_POINT('Origin',(0.,-14.320364363769,-8.26786622031554));
#77691=CARTESIAN_POINT('',(1.0466791029121,-14.5172946854278,-8.61603061885642));
#77692=CARTESIAN_POINT('',(0.,-14.5172946854278,-8.61603061885642));
#77693=CARTESIAN_POINT('',(1.27397318515336,-14.7203487384281,-8.26433068237712));
#77694=CARTESIAN_POINT('',(0.,-14.7203487384281,-8.26433068237712));
#77695=CARTESIAN_POINT('',(1.06321307504726,-14.5517058544852,-8.59418066171037));
#77696=CARTESIAN_POINT('Ctrl Pts',(1.27396816352296,-14.7203487142803,-8.2643279504713));
#77697=CARTESIAN_POINT('Ctrl Pts',(1.27358638370095,-14.7203538993621,-8.26492069772866));
#77698=CARTESIAN_POINT('Ctrl Pts',(1.27320464247765,-14.7203576752649,-8.26551344569312));
#77699=CARTESIAN_POINT('Ctrl Pts',(1.27282294197906,-14.7203600445158,-8.26610619025907));
#77700=CARTESIAN_POINT('Ctrl Pts',(1.25846331513001,-14.7204491760707,-8.28840532482972));
#77701=CARTESIAN_POINT('Ctrl Pts',(1.24415673855861,-14.7185519253579,-8.31070845907381));
#77702=CARTESIAN_POINT('Ctrl Pts',(1.23001649395264,-14.7147716059472,-8.3327942860355));
#77703=CARTESIAN_POINT('Ctrl Pts',(1.21948887965351,-14.7119571040915,-8.34923750001157));
#77704=CARTESIAN_POINT('Ctrl Pts',(1.20905339946861,-14.7080975989748,-8.3655602500653));
#77705=CARTESIAN_POINT('Ctrl Pts',(1.19876357844106,-14.7032186705677,-8.38166740526037));
#77706=CARTESIAN_POINT('Ctrl Pts',(1.1859792286154,-14.6971569589632,-8.40167936719427));
#77707=CARTESIAN_POINT('Ctrl Pts',(1.17341797868372,-14.6895218638223,-8.42136374143484));
#77708=CARTESIAN_POINT('Ctrl Pts',(1.1611939623642,-14.6803318870801,-8.44051232411174));
#77709=CARTESIAN_POINT('Ctrl Pts',(1.15084376194894,-14.6725506391983,-8.45672562612259));
#77710=CARTESIAN_POINT('Ctrl Pts',(1.14073542481799,-14.6636539606938,-8.47255474092067));
#77711=CARTESIAN_POINT('Ctrl Pts',(1.13096113608811,-14.653638573459,-8.48786193379953));
#77712=CARTESIAN_POINT('Ctrl Pts',(1.12041472380337,-14.6428320170036,-8.50437832404375));
#77713=CARTESIAN_POINT('Ctrl Pts',(1.11028262948303,-14.6307487838924,-8.52025254103047));
#77714=CARTESIAN_POINT('Ctrl Pts',(1.10069092410919,-14.6173793722391,-8.53528304214089));
#77715=CARTESIAN_POINT('Ctrl Pts',(1.09170488325421,-14.6048541669037,-8.54936444808332));
#77716=CARTESIAN_POINT('Ctrl Pts',(1.08319283673084,-14.5911996367765,-8.56270545089688));
#77717=CARTESIAN_POINT('Ctrl Pts',(1.07529796059478,-14.5763962736229,-8.57512148407864));
#77718=CARTESIAN_POINT('Ctrl Pts',(1.07108401469024,-14.5684948739734,-8.58174862949235));
#77719=CARTESIAN_POINT('Ctrl Pts',(1.06704661018399,-14.560266010431,-8.58811191638885));
#77720=CARTESIAN_POINT('Ctrl Pts',(1.06321307505127,-14.5517058544778,-8.59418066170859));
#77721=CARTESIAN_POINT('Ctrl Pts',(1.06321307506591,-14.5517058544872,-8.59418066172487));
#77722=CARTESIAN_POINT('Ctrl Pts',(1.05819043429552,-14.5404904653484,-8.60213184166998));
#77723=CARTESIAN_POINT('Ctrl Pts',(1.05264872109867,-14.5289739003893,-8.60942456847124));
#77724=CARTESIAN_POINT('Ctrl Pts',(1.0466791029121,-14.5172946854278,-8.61603061885642));
#77725=CARTESIAN_POINT('Ctrl Pts',(0.101903474593125,-14.5466088599682,
-6.23278305441235));
#77726=CARTESIAN_POINT('Ctrl Pts',(0.386418492969695,-14.5487107391251,
-7.03527911268949));
#77727=CARTESIAN_POINT('Ctrl Pts',(0.71074942397008,-14.5502903875134,-7.82193215180854));
#77728=CARTESIAN_POINT('Ctrl Pts',(1.06321307506047,-14.5517058544778,-8.59418066172874));
#77729=CARTESIAN_POINT('Ctrl Pts',(0.171922236293657,-14.6429006199952,
-6.20674945043401));
#77730=CARTESIAN_POINT('Ctrl Pts',(0.455334595134525,-14.6478634357166,
-7.00696080694915));
#77731=CARTESIAN_POINT('Ctrl Pts',(0.778555787387494,-14.652353418377,-7.79170690635246));
#77732=CARTESIAN_POINT('Ctrl Pts',(1.12978390784211,-14.6568211447152,-8.56250845780618));
#77733=CARTESIAN_POINT('Ctrl Pts',(0.285320162668475,-14.7017962883493,
-6.16544494774729));
#77734=CARTESIAN_POINT('Ctrl Pts',(0.569230210346342,-14.7088796673577,
-6.96112914568071));
#77735=CARTESIAN_POINT('Ctrl Pts',(0.892968769450175,-14.7156693678187,
-7.74177677120188));
#77736=CARTESIAN_POINT('Ctrl Pts',(1.24474780734364,-14.7225099705522,-8.50883635440985));
#77737=CARTESIAN_POINT('Ctrl Pts',(0.400000000003164,-14.7014317448243,
-6.12420321412492));
#77738=CARTESIAN_POINT('Ctrl Pts',(0.684515018379734,-14.7084242677119,
-6.91528506452676));
#77739=CARTESIAN_POINT('Ctrl Pts',(1.00884594938012,-14.7152879318301,-7.69178879550017));
#77740=CARTESIAN_POINT('Ctrl Pts',(1.36130960047051,-14.7220341995075,-8.45501116936406));
#77741=CARTESIAN_POINT('',(0.400000000003164,-14.7014317448243,-6.12420321412492));
#77742=CARTESIAN_POINT('Ctrl Pts',(1.27397005114187,-14.7203487510109,-8.26433210590187));
#77743=CARTESIAN_POINT('Ctrl Pts',(0.955180241542801,-14.7141455116759,
-7.56254390577861));
#77744=CARTESIAN_POINT('Ctrl Pts',(0.660855486066981,-14.7078427876124,
-6.8495007459751));
#77745=CARTESIAN_POINT('Ctrl Pts',(0.400000000003164,-14.7014317448243,
-6.12420321412492));
#77746=CARTESIAN_POINT('',(0.101903474593125,-14.5466088599666,-6.23278305441165));
#77747=CARTESIAN_POINT('Origin',(0.400000000003164,-14.3014473701651,-6.12773875206334));
#77748=CARTESIAN_POINT('Ctrl Pts',(0.101903474593125,-14.5466088599682,
-6.23278305441235));
#77749=CARTESIAN_POINT('Ctrl Pts',(0.386418492969695,-14.5487107391251,
-7.03527911268949));
#77750=CARTESIAN_POINT('Ctrl Pts',(0.71074942397008,-14.5502903875134,-7.82193215180854));
#77751=CARTESIAN_POINT('Ctrl Pts',(1.06321307506047,-14.5517058544778,-8.59418066172874));
#77752=CARTESIAN_POINT('Origin',(0.4,-14.2641291178216,-1.90583020886544));
#77753=CARTESIAN_POINT('Origin',(0.4,-14.3014473701651,-6.12773875205454));
#77754=CARTESIAN_POINT('',(0.4,-14.6641134924807,-1.90229467092702));
#77755=CARTESIAN_POINT('Origin',(0.4,-14.3014473701651,-6.12773875205454));
#77756=CARTESIAN_POINT('Origin',(0.4,-14.3014473701651,-6.12773875205454));
#77757=CARTESIAN_POINT('Origin',(0.,-14.7224318643355,-8.5));
#77758=CARTESIAN_POINT('',(0.4,-13.1515390292838,-9.38853550964661));
#77759=CARTESIAN_POINT('Ctrl Pts',(1.0466791029121,-14.5172946854278,-8.61603061885642));
#77760=CARTESIAN_POINT('Ctrl Pts',(0.690003264473358,-13.8194789024921,
-9.01073233783767));
#77761=CARTESIAN_POINT('Ctrl Pts',(0.4,-13.1515390292838,-9.38853550964661));
#77762=CARTESIAN_POINT('',(0.4,-10.7480230740355,-10.7480230740355));
#77763=CARTESIAN_POINT('',(0.4,-10.9666966518969,-10.6243359359852));
#77764=CARTESIAN_POINT('',(0.,-10.7480230740355,-10.7480230740355));
#77765=CARTESIAN_POINT('Origin',(0.75,0.,0.));
#77766=CARTESIAN_POINT('',(0.101903474589961,-12.6373084658892,-9.52627149865727));
#77767=CARTESIAN_POINT('Origin',(0.101903474589961,0.,0.));
#77768=CARTESIAN_POINT('Ctrl Pts',(0.400000000000002,-13.1515390292838,
-9.38853550964662));
#77769=CARTESIAN_POINT('Ctrl Pts',(0.399667068330428,-13.1507722160634,
-9.38896923800822));
#77770=CARTESIAN_POINT('Ctrl Pts',(0.399334072065998,-13.1500057038705,
-9.38940231855334));
#77771=CARTESIAN_POINT('Ctrl Pts',(0.361222357060147,-13.0623293178468,
-9.43888487823719));
#77772=CARTESIAN_POINT('Ctrl Pts',(0.317603895335242,-12.9675261252991,
-9.48627042535853));
#77773=CARTESIAN_POINT('Ctrl Pts',(0.247593608196118,-12.8350759693608,
-9.53383650224976));
#77774=CARTESIAN_POINT('Ctrl Pts',(0.22401525692456,-12.7934935689011,-9.54552407030622));
#77775=CARTESIAN_POINT('Ctrl Pts',(0.186448784436963,-12.7350850228223,
-9.55347744161429));
#77776=CARTESIAN_POINT('Ctrl Pts',(0.173696102498971,-12.7164810603858,
-9.55451281677275));
#77777=CARTESIAN_POINT('Ctrl Pts',(0.146119002493602,-12.6804794870224,
-9.55109991504693));
#77778=CARTESIAN_POINT('Ctrl Pts',(0.131473473008948,-12.6628923542562,
-9.54723530665486));
#77779=CARTESIAN_POINT('Ctrl Pts',(0.113685446200983,-12.6470179428425,
-9.53526673447708));
#77780=CARTESIAN_POINT('Ctrl Pts',(0.109816274204243,-12.6435650119036,
-9.53266338421169));
#77781=CARTESIAN_POINT('Ctrl Pts',(0.105857674425492,-12.6402842474587,
-9.5296656949327));
#77782=CARTESIAN_POINT('Ctrl Pts',(0.101903474589977,-12.6373084658893,
-9.52627149865716));
#77783=CARTESIAN_POINT('Origin',(0.4,0.,0.));
#77784=CARTESIAN_POINT('Ctrl Pts',(0.101903474589977,-12.6373084658893,
-9.52627149865717));
#77785=CARTESIAN_POINT('Ctrl Pts',(0.0695787402327775,-12.6129820907086,
-9.49852467312307));
#77786=CARTESIAN_POINT('Ctrl Pts',(0.0441999104314683,-12.5849743677384,
-9.46659930523844));
#77787=CARTESIAN_POINT('Ctrl Pts',(0.00942170958529076,-12.5242604394557,
-9.39746172821018));
#77788=CARTESIAN_POINT('Ctrl Pts',(0.000351796220688282,-12.4919792870019,
-9.36073430333122));
#77789=CARTESIAN_POINT('Ctrl Pts',(3.34461281997937E-6,-12.458775967796,
-9.3229962830415));
#77790=CARTESIAN_POINT('Ctrl Pts',(5.30031696587896E-18,-12.4581385442471,
-9.32227181813167));
#77791=CARTESIAN_POINT('Ctrl Pts',(0.,-12.4575011121161,-9.32154735742182));
#77792=CARTESIAN_POINT('Origin',(0.75,0.,0.));
#77793=CARTESIAN_POINT('Origin',(0.10190347458996,0.,-2.46519032881566E-31));
#77794=CARTESIAN_POINT('Origin',(0.4,-13.3060132833275,5.48156718273351));
#77795=CARTESIAN_POINT('Origin',(0.4,-14.2811072658456,3.82661115890556));
#77796=CARTESIAN_POINT('Origin',(0.4,0.,0.));
#77797=CARTESIAN_POINT('Origin',(0.4,-10.769766330238,-10.2761715374443));
#77798=CARTESIAN_POINT('Origin',(0.4,-10.45449610694,-10.45449610694));
#77799=CARTESIAN_POINT('Origin',(0.,-14.6820725595938,-3.93404948555832));
#77800=CARTESIAN_POINT('Origin',(0.4,10.2761715374443,-10.769766330238));
#77801=CARTESIAN_POINT('',(0.4,9.6697117559627,-12.654431433775));
#77802=CARTESIAN_POINT('',(0.4,10.6243359359852,-10.9666966518969));
#77803=CARTESIAN_POINT('Origin',(0.4,9.32154735742182,-12.4575011121161));
#77804=CARTESIAN_POINT('Origin',(0.4,10.45449610694,-10.45449610694));
#77805=CARTESIAN_POINT('Origin',(0.4,8.78256193508805,-11.4001830744621));
#77806=CARTESIAN_POINT('Origin',(0.4,12.4575011121161,-9.32154735742182));
#77807=CARTESIAN_POINT('Ctrl Pts',(0.975876659743318,8.4012251922095,-14.5513488787345));
#77808=CARTESIAN_POINT('Ctrl Pts',(0.657116047554944,8.75518920352235,-13.9356118991871));
#77809=CARTESIAN_POINT('Ctrl Pts',(0.362758547479544,9.11512949353393,-13.3092044981173));
#77810=CARTESIAN_POINT('Ctrl Pts',(0.101903474592398,9.48134128444312,-12.6710528913806));
#77811=CARTESIAN_POINT('Ctrl Pts',(1.04274635983407,8.50725783232391,-14.5764294404348));
#77812=CARTESIAN_POINT('Ctrl Pts',(0.725113127440751,8.85810731755049,-13.9604926628253));
#77813=CARTESIAN_POINT('Ctrl Pts',(0.431766345557855,9.21485636586833,-13.3343020570725));
#77814=CARTESIAN_POINT('Ctrl Pts',(0.171922236292934,9.57774919679076,-12.6966530089968));
#77815=CARTESIAN_POINT('Ctrl Pts',(1.15757519551698,8.59000236282895,-14.5633115305157));
#77816=CARTESIAN_POINT('Ctrl Pts',(0.8394387387802,8.93723219358694,-13.9493126912418));
#77817=CARTESIAN_POINT('Ctrl Pts',(0.545620573531762,9.29027284840102,-13.3253566536154));
#77818=CARTESIAN_POINT('Ctrl Pts',(0.285320162667751,9.64940659310159,-12.6903300945564));
#77819=CARTESIAN_POINT('Ctrl Pts',(1.27397318515336,8.61603061885642,-14.5172946854278));
#77820=CARTESIAN_POINT('Ctrl Pts',(0.955212572964985,8.96154828660087,-13.9064342046133));
#77821=CARTESIAN_POINT('Ctrl Pts',(0.660855072889585,9.31261568156926,-13.2857620430748));
#77822=CARTESIAN_POINT('Ctrl Pts',(0.400000000002439,9.66971175595937,-12.6544314337809));
#77823=CARTESIAN_POINT('',(0.101903474592399,9.48134128444231,-12.6710528913795));
#77824=CARTESIAN_POINT('Origin',(0.400000000002438,9.32154735741848,-12.457501112122));
#77825=CARTESIAN_POINT('',(1.27397318515336,8.61603061885642,-14.5172946854278));
#77826=CARTESIAN_POINT('Ctrl Pts',(0.400000000002439,9.66971175595937,-12.6544314337809));
#77827=CARTESIAN_POINT('Ctrl Pts',(0.660855072889585,9.31261568156926,-13.2857620430748));
#77828=CARTESIAN_POINT('Ctrl Pts',(0.955212572964985,8.96154828660087,-13.9064342046133));
#77829=CARTESIAN_POINT('Ctrl Pts',(1.27397318515336,8.61603061885642,-14.5172946854278));
#77830=CARTESIAN_POINT('',(0.975876659743319,8.40122519220951,-14.5513488787345));
#77831=CARTESIAN_POINT('Origin',(1.27397318515336,8.26786622031554,-14.320364363769));
#77832=CARTESIAN_POINT('Ctrl Pts',(0.975876659743318,8.4012251922095,-14.5513488787345));
#77833=CARTESIAN_POINT('Ctrl Pts',(0.657116047554944,8.75518920352235,-13.9356118991871));
#77834=CARTESIAN_POINT('Ctrl Pts',(0.362758547479544,9.11512949353393,-13.3092044981173));
#77835=CARTESIAN_POINT('Ctrl Pts',(0.101903474592398,9.48134128444312,-12.6710528913806));
#77836=CARTESIAN_POINT('Origin',(1.27397318515336,8.26786622031554,-14.320364363769));
#77837=CARTESIAN_POINT('',(1.27397318515336,8.26433068237712,-14.7203487384281));
#77838=CARTESIAN_POINT('Origin',(1.27397318515336,8.26786622031554,-14.320364363769));
#77839=CARTESIAN_POINT('Origin',(1.27397318515336,8.26786622031554,-14.320364363769));
#77840=CARTESIAN_POINT('Origin',(0.4,9.32154735741685,-12.4575011121198));
#77841=CARTESIAN_POINT('Origin',(0.4,9.32154735741685,-12.4575011121198));
#77842=CARTESIAN_POINT('Origin',(0.4,12.4575011121161,-9.32154735742182));
#77843=CARTESIAN_POINT('Origin',(0.,14.7224318643355,-8.50000000000001));
#77844=CARTESIAN_POINT('',(0.,14.6820725595938,-3.93404948555831));
#77845=CARTESIAN_POINT('Origin',(0.4,0.,0.));
#77846=CARTESIAN_POINT('',(0.101903474593116,6.23278305441163,-14.5466088599666));
#77847=CARTESIAN_POINT('Origin',(0.10190347458996,-5.55111512312578E-16,
-1.11022302462516E-15));
#77848=CARTESIAN_POINT('Origin',(0.4,6.12773875205454,-14.3014473701651));
#77849=CARTESIAN_POINT('Origin',(0.75,0.,0.));
#77850=CARTESIAN_POINT('Ctrl Pts',(0.101903474593116,6.23278305441232,-14.5466088599682));
#77851=CARTESIAN_POINT('Ctrl Pts',(0.36275843270851,6.9685441290442,-14.5485359483959));
#77852=CARTESIAN_POINT('Ctrl Pts',(0.657121506632204,7.69101148350598,-14.5500222375035));
#77853=CARTESIAN_POINT('Ctrl Pts',(0.975876659743319,8.40122519220951,-14.5513488787345));
#77854=CARTESIAN_POINT('Origin',(0.,8.26786622031554,-14.320364363769));
#77855=CARTESIAN_POINT('',(0.,8.61603061885642,-14.5172946854278));
#77856=CARTESIAN_POINT('',(0.,8.26433068237712,-14.7203487384281));
#77857=CARTESIAN_POINT('Ctrl Pts',(0.101903474593116,6.23278305441232,-14.5466088599682));
#77858=CARTESIAN_POINT('Ctrl Pts',(0.36275843270851,6.9685441290442,-14.5485359483959));
#77859=CARTESIAN_POINT('Ctrl Pts',(0.657121506632204,7.69101148350598,-14.5500222375035));
#77860=CARTESIAN_POINT('Ctrl Pts',(0.975876659743319,8.40122519220951,-14.5513488787345));
#77861=CARTESIAN_POINT('Ctrl Pts',(0.171922236293649,6.20674945043399,-14.6429006199952));
#77862=CARTESIAN_POINT('Ctrl Pts',(0.431766231231625,6.94041581742676,-14.647450731601));
#77863=CARTESIAN_POINT('Ctrl Pts',(0.725118567210565,7.6610997761619,-14.6515923684846));
#77864=CARTESIAN_POINT('Ctrl Pts',(1.04274635983407,8.36992927572594,-14.655716119554));
#77865=CARTESIAN_POINT('Ctrl Pts',(0.285320162668467,6.16544494774726,-14.7017962883493));
#77866=CARTESIAN_POINT('Ctrl Pts',(0.545620459004768,6.8949606313457,-14.7082906187544));
#77867=CARTESIAN_POINT('Ctrl Pts',(0.839444187168207,7.61185513900119,-14.7145265725021));
#77868=CARTESIAN_POINT('Ctrl Pts',(1.15757519551698,8.31719656723893,-14.7208160300361));
#77869=CARTESIAN_POINT('Ctrl Pts',(0.400000000003156,6.1242032141249,-14.7014317448243));
#77870=CARTESIAN_POINT('Ctrl Pts',(0.66085495811855,6.84949927803705,-14.707842774637));
#77871=CARTESIAN_POINT('Ctrl Pts',(0.955218032042244,7.56256317259036,-14.714145681979));
#77872=CARTESIAN_POINT('Ctrl Pts',(1.27397318515336,8.26433068237712,-14.7203487384281));
#77873=CARTESIAN_POINT('',(0.400000000003156,6.1242032141249,-14.7014317448243));
#77874=CARTESIAN_POINT('Ctrl Pts',(1.27397318515336,8.26433068237712,-14.7203487384281));
#77875=CARTESIAN_POINT('Ctrl Pts',(0.955218032042244,7.56256317259036,-14.714145681979));
#77876=CARTESIAN_POINT('Ctrl Pts',(0.66085495811855,6.84949927803705,-14.707842774637));
#77877=CARTESIAN_POINT('Ctrl Pts',(0.400000000003156,6.1242032141249,-14.7014317448243));
#77878=CARTESIAN_POINT('Origin',(0.400000000003156,6.12773875206332,-14.3014473701651));
#77879=CARTESIAN_POINT('Origin',(0.4,3.51454243995435,-14.4649770035306));
#77880=CARTESIAN_POINT('',(0.4,3.93404948555831,-14.6820725595938));
#77881=CARTESIAN_POINT('',(0.4,2.04700031104924,-15.7939149700788));
#77882=CARTESIAN_POINT('',(0.4,3.71759649295465,-14.8096058641331));
#77883=CARTESIAN_POINT('Origin',(0.4,1.84394625804894,-15.4492861094764));
#77884=CARTESIAN_POINT('Origin',(0.4,3.82661115890556,-14.2811072658456));
#77885=CARTESIAN_POINT('Origin',(0.4,1.90583020886544,-14.2641291178216));
#77886=CARTESIAN_POINT('Origin',(0.4,6.12773875205454,-14.3014473701651));
#77887=CARTESIAN_POINT('',(0.4,1.90229467092702,-14.6641134924807));
#77888=CARTESIAN_POINT('Origin',(1.27397318515331,-2.77555756156289E-15,
-16.5357324406311));
#77889=CARTESIAN_POINT('',(1.27397318218458,0.203054053000297,-16.8803613012335));
#77890=CARTESIAN_POINT('',(0.975876659743315,-2.15105711021124E-15,-16.802450384419));
#77891=CARTESIAN_POINT('Origin',(1.27397318341511,3.29726905501371E-9,-16.5357324386883));
#77892=CARTESIAN_POINT('',(1.27397318515333,-0.203054053000348,-16.8803613012335));
#77893=CARTESIAN_POINT('Origin',(1.27397318515331,-2.77555756156289E-15,
-16.5357324406311));
#77894=CARTESIAN_POINT('Origin',(1.27397318515336,-2.56739074444567E-15,
-16.5357324406311));
#77895=CARTESIAN_POINT('Origin',(0.,-2.77555756156289E-15,-16.5357324406311));
#77896=CARTESIAN_POINT('',(0.,-0.203054053000303,-16.8803613012335));
#77897=CARTESIAN_POINT('',(0.,0.203054053000297,-16.8803613012335));
#77898=CARTESIAN_POINT('Ctrl Pts',(0.101903474593096,-1.87555596858592,
-15.7141243388544));
#77899=CARTESIAN_POINT('Ctrl Pts',(0.362757933509743,-1.23933294859665,
-16.0836730764964));
#77900=CARTESIAN_POINT('Ctrl Pts',(0.65712213971653,-0.614398572969214,
-16.4461953326244));
#77901=CARTESIAN_POINT('Ctrl Pts',(0.975876659743316,-2.28983498828939E-15,
-16.802450384419));
#77902=CARTESIAN_POINT('Ctrl Pts',(0.171922236293629,-1.94624761099671,
-15.7844986472237));
#77903=CARTESIAN_POINT('Ctrl Pts',(0.43176573396754,-1.31315016664401,-16.1552716334103));
#77904=CARTESIAN_POINT('Ctrl Pts',(0.725119198055823,-0.691087942048844,
-16.5192017960841));
#77905=CARTESIAN_POINT('Ctrl Pts',(1.04274635983407,-0.0792866791192692,
-16.8771871080498));
#77906=CARTESIAN_POINT('Ctrl Pts',(0.285320162668447,-2.01146619379113,
-15.8148515408478));
#77907=CARTESIAN_POINT('Ctrl Pts',(0.545619960867456,-1.38293544736135,
-16.1852329289574));
#77908=CARTESIAN_POINT('Ctrl Pts',(0.83944481901291,-0.765202158989165,
-16.5490820972111));
#77909=CARTESIAN_POINT('Ctrl Pts',(1.15757519551697,-0.157504499520388,
-16.9071989300679));
#77910=CARTESIAN_POINT('Ctrl Pts',(0.400000000003136,-2.04700031104173,
-15.7939149700833));
#77911=CARTESIAN_POINT('Ctrl Pts',(0.66085445891978,-1.42208220524482,-16.162114412096));
#77912=CARTESIAN_POINT('Ctrl Pts',(0.95521866512657,-0.807699814903305,
-16.5241062494389));
#77913=CARTESIAN_POINT('Ctrl Pts',(1.27397318515336,-0.203054053000302,
-16.8803613012335));
#77914=CARTESIAN_POINT('',(0.400000000003136,-2.04700031104173,-15.7939149700833));
#77915=CARTESIAN_POINT('Ctrl Pts',(1.27397318515336,-0.203054053000302,
-16.8803613012335));
#77916=CARTESIAN_POINT('Ctrl Pts',(0.95521866512657,-0.807699814903305,
-16.5241062494389));
#77917=CARTESIAN_POINT('Ctrl Pts',(0.66085445891978,-1.42208220524482,-16.162114412096));
#77918=CARTESIAN_POINT('Ctrl Pts',(0.400000000003136,-2.04700031104173,
-15.7939149700833));
#77919=CARTESIAN_POINT('',(0.101903474593097,-1.87555596858571,-15.7141243388527));
#77920=CARTESIAN_POINT('Origin',(0.400000000003136,-1.84394625804143,-15.4492861094808));
#77921=CARTESIAN_POINT('Ctrl Pts',(0.101903474593096,-1.87555596858592,
-15.7141243388544));
#77922=CARTESIAN_POINT('Ctrl Pts',(0.362757933509743,-1.23933294859665,
-16.0836730764964));
#77923=CARTESIAN_POINT('Ctrl Pts',(0.65712213971653,-0.614398572969214,
-16.4461953326244));
#77924=CARTESIAN_POINT('Ctrl Pts',(0.975876659743316,-2.28983498828939E-15,
-16.802450384419));
#77925=CARTESIAN_POINT('Ctrl Pts',(0.975876659743315,-1.45716771982052E-15,
-16.802450384419));
#77926=CARTESIAN_POINT('Ctrl Pts',(0.657122139716523,0.614398572969222,
-16.4461953326244));
#77927=CARTESIAN_POINT('Ctrl Pts',(0.362757933509742,1.23933294859665,-16.0836730764964));
#77928=CARTESIAN_POINT('Ctrl Pts',(0.101903474593097,1.87555596858592,-15.7141243388544));
#77929=CARTESIAN_POINT('Ctrl Pts',(1.04274635983406,0.0792866791192654,
-16.8771871080498));
#77930=CARTESIAN_POINT('Ctrl Pts',(0.725119198055816,0.691087942048852,
-16.5192017960841));
#77931=CARTESIAN_POINT('Ctrl Pts',(0.431765733967538,1.31315016664401,-16.1552716334103));
#77932=CARTESIAN_POINT('Ctrl Pts',(0.17192223629363,1.94624761099671,-15.7844986472237));
#77933=CARTESIAN_POINT('Ctrl Pts',(1.15757519551697,0.157504499520384,-16.9071989300679));
#77934=CARTESIAN_POINT('Ctrl Pts',(0.839444819012904,0.765202158989172,
-16.5490820972111));
#77935=CARTESIAN_POINT('Ctrl Pts',(0.545619960867455,1.38293544736135,-16.1852329289574));
#77936=CARTESIAN_POINT('Ctrl Pts',(0.285320162668447,2.01146619379112,-15.8148515408478));
#77937=CARTESIAN_POINT('Ctrl Pts',(1.27397318515336,0.203054053000298,-16.8803613012335));
#77938=CARTESIAN_POINT('Ctrl Pts',(0.955218665126563,0.807699814903313,
-16.5241062494389));
#77939=CARTESIAN_POINT('Ctrl Pts',(0.660854458919779,1.42208220524482,-16.162114412096));
#77940=CARTESIAN_POINT('Ctrl Pts',(0.400000000003137,2.04700031104172,-15.7939149700833));
#77941=CARTESIAN_POINT('',(0.101903474593097,1.87555596858571,-15.7141243388527));
#77942=CARTESIAN_POINT('Ctrl Pts',(0.975876659743315,-1.45716771982052E-15,
-16.802450384419));
#77943=CARTESIAN_POINT('Ctrl Pts',(0.657122139716523,0.614398572969222,
-16.4461953326244));
#77944=CARTESIAN_POINT('Ctrl Pts',(0.362757933509742,1.23933294859665,-16.0836730764964));
#77945=CARTESIAN_POINT('Ctrl Pts',(0.101903474593097,1.87555596858592,-15.7141243388544));
#77946=CARTESIAN_POINT('Origin',(0.400000000003137,1.84394625804142,-15.4492861094808));
#77947=CARTESIAN_POINT('Ctrl Pts',(0.400000000003137,2.04700031104172,-15.7939149700833));
#77948=CARTESIAN_POINT('Ctrl Pts',(0.660854458781283,1.42208220557661,-16.1621144119006));
#77949=CARTESIAN_POINT('Ctrl Pts',(0.955218664813989,0.807699815555703,
-16.5241062490545));
#77950=CARTESIAN_POINT('Ctrl Pts',(1.27397318464564,0.203054053963375,-16.8803613006661));
#77951=CARTESIAN_POINT('Origin',(0.4,-4.18880546608629,-14.2843087701924));
#77952=CARTESIAN_POINT('',(0.4,-3.93404948555831,-14.6820725595938));
#77953=CARTESIAN_POINT('',(0.4,-6.12420321411612,-14.7014317448242));
#77954=CARTESIAN_POINT('',(0.4,-4.18526992814787,-14.6842931448515));
#77955=CARTESIAN_POINT('Origin',(0.4,-6.12773875205454,-14.3014473701651));
#77956=CARTESIAN_POINT('Origin',(0.4,-3.82661115890556,-14.2811072658456));
#77957=CARTESIAN_POINT('Origin',(0.4,-5.48156718273351,-13.3060132833275));
#77958=CARTESIAN_POINT('Origin',(0.4,-1.84394625804895,-15.4492861094764));
#77959=CARTESIAN_POINT('',(0.4,-5.68462123573381,-13.65064214393));
#77960=CARTESIAN_POINT('Origin',(1.27397318515333,-8.26786622031554,-14.320364363769));
#77961=CARTESIAN_POINT('',(1.27397318515336,-8.26433068237712,-14.7203487384281));
#77962=CARTESIAN_POINT('',(0.975876659743318,-8.40122519220951,-14.5513488787345));
#77963=CARTESIAN_POINT('Origin',(1.27397318515336,-8.26786622031554,-14.320364363769));
#77964=CARTESIAN_POINT('',(1.27397318515334,-8.61603061885645,-14.5172946854278));
#77965=CARTESIAN_POINT('Origin',(1.27397318515333,-8.26786622031554,-14.320364363769));
#77966=CARTESIAN_POINT('Origin',(1.27397318515336,-8.26786622031554,-14.320364363769));
#77967=CARTESIAN_POINT('Origin',(0.,-8.26786622031554,-14.320364363769));
#77968=CARTESIAN_POINT('',(0.,-8.61603061885643,-14.5172946854278));
#77969=CARTESIAN_POINT('',(0.,-8.26433068237712,-14.7203487384281));
#77970=CARTESIAN_POINT('Ctrl Pts',(0.101903474593114,-9.48134128444212,
-12.6710528913823));
#77971=CARTESIAN_POINT('Ctrl Pts',(0.362758167198483,-9.11513002740676,
-13.3092035678037));
#77972=CARTESIAN_POINT('Ctrl Pts',(0.657121637769335,-8.75518299593385,
-13.9356226975781));
#77973=CARTESIAN_POINT('Ctrl Pts',(0.975876659743318,-8.40122519220951,
-14.5513488787345));
#77974=CARTESIAN_POINT('Ctrl Pts',(0.171922236293647,-9.57774919678977,
-12.6966530089985));
#77975=CARTESIAN_POINT('Ctrl Pts',(0.431765966750601,-9.21485689490269,
-13.3343011274915));
#77976=CARTESIAN_POINT('Ctrl Pts',(0.725118697883895,-8.8581011645825,-13.9605034647202));
#77977=CARTESIAN_POINT('Ctrl Pts',(1.04274635983407,-8.50725783232392,-14.5764294404347));
#77978=CARTESIAN_POINT('Ctrl Pts',(0.285320162668464,-9.64940659310061,
-12.6903300945582));
#77979=CARTESIAN_POINT('Ctrl Pts',(0.5456201940593,-9.29027337195529,-13.3253557278576));
#77980=CARTESIAN_POINT('Ctrl Pts',(0.839444318048562,-8.93722610409809,
-13.9493234591504));
#77981=CARTESIAN_POINT('Ctrl Pts',(1.15757519551698,-8.59000236282895,-14.5633115305157));
#77982=CARTESIAN_POINT('Ctrl Pts',(0.400000000003154,-9.66971175595839,
-12.6544314337826));
#77983=CARTESIAN_POINT('Ctrl Pts',(0.660854692608521,-9.31261620215297,
-13.2857611227051));
#77984=CARTESIAN_POINT('Ctrl Pts',(0.955218163179375,-8.9615422271388,-13.9064449174835));
#77985=CARTESIAN_POINT('Ctrl Pts',(1.27397318515336,-8.61603061885642,-14.5172946854278));
#77986=CARTESIAN_POINT('',(0.400000000003154,-9.66971175595839,-12.6544314337826));
#77987=CARTESIAN_POINT('Ctrl Pts',(1.27397318515336,-8.61603061885642,-14.5172946854278));
#77988=CARTESIAN_POINT('Ctrl Pts',(0.955218163179375,-8.9615422271388,-13.9064449174835));
#77989=CARTESIAN_POINT('Ctrl Pts',(0.660854692608521,-9.31261620215297,
-13.2857611227051));
#77990=CARTESIAN_POINT('Ctrl Pts',(0.400000000003154,-9.66971175595839,
-12.6544314337826));
#77991=CARTESIAN_POINT('',(0.101903474593115,-9.48134128444107,-12.6710528913809));
#77992=CARTESIAN_POINT('Origin',(0.400000000003154,-9.32154735741751,-12.4575011121237));
#77993=CARTESIAN_POINT('Ctrl Pts',(0.101903474593114,-9.48134128444212,
-12.6710528913823));
#77994=CARTESIAN_POINT('Ctrl Pts',(0.362758167198483,-9.11513002740676,
-13.3092035678037));
#77995=CARTESIAN_POINT('Ctrl Pts',(0.657121637769335,-8.75518299593385,
-13.9356226975781));
#77996=CARTESIAN_POINT('Ctrl Pts',(0.975876659743318,-8.40122519220951,
-14.5513488787345));
#77997=CARTESIAN_POINT('Ctrl Pts',(0.975876659743318,-8.40122519220951,
-14.5513488787345));
#77998=CARTESIAN_POINT('Ctrl Pts',(0.657121506632204,-7.69101148350598,
-14.5500222375035));
#77999=CARTESIAN_POINT('Ctrl Pts',(0.362758432708511,-6.96854412904421,
-14.5485359483959));
#78000=CARTESIAN_POINT('Ctrl Pts',(0.101903474593118,-6.23278305441233,
-14.5466088599682));
#78001=CARTESIAN_POINT('Ctrl Pts',(1.04274635983407,-8.36992927572594,-14.655716119554));
#78002=CARTESIAN_POINT('Ctrl Pts',(0.725118567210564,-7.6610997761619,-14.6515923684846));
#78003=CARTESIAN_POINT('Ctrl Pts',(0.431766231231625,-6.94041581742676,
-14.647450731601));
#78004=CARTESIAN_POINT('Ctrl Pts',(0.171922236293651,-6.206749450434,-14.6429006199952));
#78005=CARTESIAN_POINT('Ctrl Pts',(1.15757519551698,-8.31719656723894,-14.7208160300361));
#78006=CARTESIAN_POINT('Ctrl Pts',(0.839444187168207,-7.61185513900119,
-14.7145265725021));
#78007=CARTESIAN_POINT('Ctrl Pts',(0.545620459004768,-6.89496063134571,
-14.7082906187544));
#78008=CARTESIAN_POINT('Ctrl Pts',(0.285320162668469,-6.16544494774728,
-14.7017962883493));
#78009=CARTESIAN_POINT('Ctrl Pts',(1.27397318515336,-8.26433068237712,-14.7203487384281));
#78010=CARTESIAN_POINT('Ctrl Pts',(0.955218032042244,-7.56256317259036,
-14.714145681979));
#78011=CARTESIAN_POINT('Ctrl Pts',(0.660854958118549,-6.84949927803706,
-14.707842774637));
#78012=CARTESIAN_POINT('Ctrl Pts',(0.400000000003158,-6.12420321412491,
-14.7014317448243));
#78013=CARTESIAN_POINT('',(0.10190347459312,-6.23278305441164,-14.5466088599666));
#78014=CARTESIAN_POINT('Ctrl Pts',(0.975876659743318,-8.40122519220951,
-14.5513488787345));
#78015=CARTESIAN_POINT('Ctrl Pts',(0.657121506632204,-7.69101148350598,
-14.5500222375035));
#78016=CARTESIAN_POINT('Ctrl Pts',(0.362758432708511,-6.96854412904421,
-14.5485359483959));
#78017=CARTESIAN_POINT('Ctrl Pts',(0.101903474593118,-6.23278305441233,
-14.5466088599682));
#78018=CARTESIAN_POINT('Origin',(0.400000000003158,-6.12773875206333,-14.3014473701651));
#78019=CARTESIAN_POINT('Ctrl Pts',(0.400000000003158,-6.12420321412491,
-14.7014317448243));
#78020=CARTESIAN_POINT('Ctrl Pts',(0.660854958118549,-6.84949927803706,
-14.707842774637));
#78021=CARTESIAN_POINT('Ctrl Pts',(0.955218032042244,-7.56256317259036,
-14.714145681979));
#78022=CARTESIAN_POINT('Ctrl Pts',(1.27397318515336,-8.26433068237712,-14.7203487384281));
#78023=CARTESIAN_POINT('Origin',(0.4,-11.4001830744621,-8.78256193508805));
#78024=CARTESIAN_POINT('Origin',(0.4,-9.32154735742183,-12.4575011121161));
#78025=CARTESIAN_POINT('',(0.4,-11.748347473003,-8.97949225674692));
#78026=CARTESIAN_POINT('Origin',(0.4,-9.32154735742182,-12.4575011121161));
#78027=CARTESIAN_POINT('Origin',(0.4,-9.32154735742182,-12.4575011121161));
#78028=CARTESIAN_POINT('Origin',(0.4,-6.12773875206194,-14.3014473701619));
#78029=CARTESIAN_POINT('Origin',(0.4,-6.12773875206194,-14.3014473701619));
#78030=CARTESIAN_POINT('Origin',(0.4,-1.84394625804895,-15.4492861094764));
#78031=CARTESIAN_POINT('Origin',(0.4,-1.84394625804895,-15.4492861094764));
#78032=CARTESIAN_POINT('Origin',(0.4,1.843946258041,-15.4492861094773));
#78033=CARTESIAN_POINT('Origin',(0.4,1.843946258041,-15.4492861094773));
#78034=CARTESIAN_POINT('Origin',(0.4,6.12773875205454,-14.3014473701651));
#78035=CARTESIAN_POINT('Origin',(0.,8.5,-14.7224318643355));
#78036=CARTESIAN_POINT('Origin',(0.75,0.,0.));
#78037=CARTESIAN_POINT('Origin',(0.10190347458996,-7.87958859913272E-16,
0.));
#78038=CARTESIAN_POINT('Origin',(0.4,0.,0.));
#78039=CARTESIAN_POINT('Origin',(0.75,0.,0.));
#78040=CARTESIAN_POINT('Origin',(0.101903474589959,-5.55111512312578E-16,
0.));
#78041=CARTESIAN_POINT('Origin',(0.4,0.,0.));
#78042=CARTESIAN_POINT('Origin',(0.,-10.7480230740355,-10.7480230740355));
#78043=CARTESIAN_POINT('Origin',(0.,-3.93404948555831,-14.6820725595938));
#78044=CARTESIAN_POINT('',(0.,-3.93404948555831,-14.6820725595938));
#78045=CARTESIAN_POINT('Origin',(0.,3.93404948555831,-14.6820725595938));
#78046=CARTESIAN_POINT('',(0.,3.93404948555831,-14.6820725595938));
#78047=CARTESIAN_POINT('Origin',(0.4,-14.2843087701924,4.18880546608627));
#78048=CARTESIAN_POINT('Origin',(0.4,-14.3014473701652,6.12773875207098));
#78049=CARTESIAN_POINT('Origin',(0.400000000005235,-14.3014473701652,6.1277387520691));
#78050=CARTESIAN_POINT('Origin',(0.4,0.,0.));
#78051=CARTESIAN_POINT('Origin',(0.4,-1.48088984913629E-15,12.0923832909811));
#78052=CARTESIAN_POINT('Origin',(0.4,0.,0.));
#78053=CARTESIAN_POINT('Origin',(0.101903474589959,-5.55111512312578E-16,
0.));
#78054=CARTESIAN_POINT('Origin',(0.,-3.93404948555832,14.6820725595938));
#78055=CARTESIAN_POINT('',(0.4,-3.93404948555832,14.6820725595938));
#78056=CARTESIAN_POINT('',(0.,-3.93404948555832,14.6820725595938));
#78057=CARTESIAN_POINT('Origin',(0.4,-3.1577284155994,14.6752105100511));
#78058=CARTESIAN_POINT('Origin',(0.75,0.,0.));
#78059=CARTESIAN_POINT('Origin',(1.27397318515336,1.04083408558608E-15,
16.5357324406311));
#78060=CARTESIAN_POINT('',(1.27397318515336,-0.203054053000298,16.8803613012335));
#78061=CARTESIAN_POINT('',(1.27397318515336,0.203054053000301,16.8803613012335));
#78062=CARTESIAN_POINT('Origin',(1.27397318515336,1.04083408558608E-15,
16.5357324406311));
#78063=CARTESIAN_POINT('',(0.975876659743317,3.46944695195361E-16,16.802450384419));
#78064=CARTESIAN_POINT('Origin',(1.27397318515336,1.04083408558608E-15,
16.5357324406311));
#78065=CARTESIAN_POINT('Origin',(1.27397318515336,1.04083408558608E-15,
16.5357324406311));
#78066=CARTESIAN_POINT('Origin',(0.,8.32667268468867E-16,16.5357324406311));
#78067=CARTESIAN_POINT('',(0.,-0.203054053000299,16.8803613012335));
#78068=CARTESIAN_POINT('',(0.,0.203054053000301,16.8803613012335));
#78069=CARTESIAN_POINT('Origin',(0.,1.04094977927525E-15,17.));
#78070=CARTESIAN_POINT('',(0.400000000003121,-2.04700031103429,15.7939149700876));
#78071=CARTESIAN_POINT('Ctrl Pts',(0.400000000000002,-2.04700031104923,
15.7939149700788));
#78072=CARTESIAN_POINT('Ctrl Pts',(0.660849039304145,-1.42209518879036,
16.1621067622389));
#78073=CARTESIAN_POINT('Ctrl Pts',(0.955212095439956,-0.807712276948292,
16.524098906848));
#78074=CARTESIAN_POINT('Ctrl Pts',(1.27397318515336,-0.203054053000297,
16.8803613012335));
#78075=CARTESIAN_POINT('',(0.4,-3.71759649295465,14.8096058641331));
#78076=CARTESIAN_POINT('Ctrl Pts',(0.975876659743318,2.28983498828939E-15,
16.802450384419));
#78077=CARTESIAN_POINT('Ctrl Pts',(0.657115570029917,-0.614411236024409,
16.4461879900334));
#78078=CARTESIAN_POINT('Ctrl Pts',(0.362752513894104,-1.23934616701756,
16.0836653986058));
#78079=CARTESIAN_POINT('Ctrl Pts',(0.101903474589961,-1.87555596859357,
15.71412433885));
#78080=CARTESIAN_POINT('Ctrl Pts',(1.04274635983407,-0.0792866791192643,
16.8771871080498));
#78081=CARTESIAN_POINT('Ctrl Pts',(0.725112651604614,-0.69110055157221,
16.5191944178317));
#78082=CARTESIAN_POINT('Ctrl Pts',(0.431760335356032,-1.31316332012672,
16.1552639300842));
#78083=CARTESIAN_POINT('Ctrl Pts',(0.171922236290506,-1.94624761100432,
15.7844986472193));
#78084=CARTESIAN_POINT('Ctrl Pts',(1.15757519551698,-0.157504499520383,
16.9071989300679));
#78085=CARTESIAN_POINT('Ctrl Pts',(0.8394382621902,-0.765214683935252,16.549074716248));
#78086=CARTESIAN_POINT('Ctrl Pts',(0.545614552775671,-1.38294850596453,
16.1852252337673));
#78087=CARTESIAN_POINT('Ctrl Pts',(0.285320162665319,-2.01146619379868,
15.8148515408434));
#78088=CARTESIAN_POINT('Ctrl Pts',(1.27397318515336,-0.203054053000297,
16.8803613012335));
#78089=CARTESIAN_POINT('Ctrl Pts',(0.955212095439956,-0.807712276948292,
16.524098906848));
#78090=CARTESIAN_POINT('Ctrl Pts',(0.660849039304145,-1.42209518879036,
16.1621067622389));
#78091=CARTESIAN_POINT('Ctrl Pts',(0.400000000000002,-2.04700031104923,
15.7939149700788));
#78092=CARTESIAN_POINT('',(0.101903474589964,-1.87555596859356,15.71412433885));
#78093=CARTESIAN_POINT('Ctrl Pts',(0.975876659743318,2.28983498828939E-15,
16.802450384419));
#78094=CARTESIAN_POINT('Ctrl Pts',(0.657115570029917,-0.614411236024409,
16.4461879900334));
#78095=CARTESIAN_POINT('Ctrl Pts',(0.362752513894104,-1.23934616701756,
16.0836653986058));
#78096=CARTESIAN_POINT('Ctrl Pts',(0.101903474589961,-1.87555596859357,
15.71412433885));
#78097=CARTESIAN_POINT('Origin',(0.400000000000001,-1.84394625804893,15.4492861094764));
#78098=CARTESIAN_POINT('Ctrl Pts',(0.101903474589961,1.87555596859357,15.71412433885));
#78099=CARTESIAN_POINT('Ctrl Pts',(0.362752280919966,1.23934673524058,16.0836650685547));
#78100=CARTESIAN_POINT('Ctrl Pts',(0.657115315847402,0.614411725960595,
16.4461877059471));
#78101=CARTESIAN_POINT('Ctrl Pts',(0.975876659743317,2.08166817117217E-16,
16.802450384419));
#78102=CARTESIAN_POINT('Ctrl Pts',(0.171922236290506,1.94624761100432,15.7844986472193));
#78103=CARTESIAN_POINT('Ctrl Pts',(0.431760103284805,1.31316388555823,16.1552635989397));
#78104=CARTESIAN_POINT('Ctrl Pts',(0.725112398321083,0.691101039437237,
16.5191941323656));
#78105=CARTESIAN_POINT('Ctrl Pts',(1.04274635983407,0.0792866791192671,
16.8771871080498));
#78106=CARTESIAN_POINT('Ctrl Pts',(0.285320162665318,2.01146619379868,15.8148515408434));
#78107=CARTESIAN_POINT('Ctrl Pts',(0.545614320296911,1.38294906731744,16.1852249029725));
#78108=CARTESIAN_POINT('Ctrl Pts',(0.839438008505393,0.76521516852797,16.549074430677));
#78109=CARTESIAN_POINT('Ctrl Pts',(1.15757519551698,0.157504499520386,16.9071989300679));
#78110=CARTESIAN_POINT('Ctrl Pts',(0.400000000000001,2.04700031104923,15.7939149700788));
#78111=CARTESIAN_POINT('Ctrl Pts',(0.660848806330008,1.42209574691674,16.1621064333929));
#78112=CARTESIAN_POINT('Ctrl Pts',(0.955211841257442,0.807712759107352,
16.5240986227616));
#78113=CARTESIAN_POINT('Ctrl Pts',(1.27397318515336,0.2030540530003,16.8803613012335));
#78114=CARTESIAN_POINT('',(0.40000000000328,2.04700031103352,15.7939149700881));
#78115=CARTESIAN_POINT('Ctrl Pts',(1.27397318515336,0.2030540530003,16.8803613012335));
#78116=CARTESIAN_POINT('Ctrl Pts',(0.955211841257442,0.807712759107352,
16.5240986227616));
#78117=CARTESIAN_POINT('Ctrl Pts',(0.660848806330008,1.42209574691674,16.1621064333929));
#78118=CARTESIAN_POINT('Ctrl Pts',(0.400000000000001,2.04700031104923,15.7939149700788));
#78119=CARTESIAN_POINT('',(0.101903474589964,1.87555596859356,15.71412433885));
#78120=CARTESIAN_POINT('Origin',(0.400000000000002,1.84394625804893,15.4492861094764));
#78121=CARTESIAN_POINT('Ctrl Pts',(0.101903474589961,1.87555596859357,15.71412433885));
#78122=CARTESIAN_POINT('Ctrl Pts',(0.362752280919966,1.23934673524058,16.0836650685547));
#78123=CARTESIAN_POINT('Ctrl Pts',(0.657115315847402,0.614411725960595,
16.4461877059471));
#78124=CARTESIAN_POINT('Ctrl Pts',(0.975876659743317,2.08166817117217E-16,
16.802450384419));
#78125=CARTESIAN_POINT('Origin',(0.4,5.48156718273351,13.3060132833275));
#78126=CARTESIAN_POINT('Origin',(0.4,1.84394625803322,15.4492861094856));
#78127=CARTESIAN_POINT('',(0.4,3.93404948555832,14.6820725595938));
#78128=CARTESIAN_POINT('',(0.4,5.68462123573381,13.65064214393));
#78129=CARTESIAN_POINT('Origin',(0.4,3.82661115890557,14.2811072658456));
#78130=CARTESIAN_POINT('Origin',(0.4,0.,0.));
#78131=CARTESIAN_POINT('Origin',(0.4,-1.84394625804893,15.4492861094764));
#78132=CARTESIAN_POINT('Origin',(0.10190347458996,-7.87958859913274E-16,
0.));
#78133=CARTESIAN_POINT('Origin',(0.4,1.84394625804893,15.4492861094764));
#78134=CARTESIAN_POINT('Origin',(0.400000000000002,1.84394625804893,15.4492861094764));
#78135=CARTESIAN_POINT('Origin',(0.4,-3.51454243995435,14.4649770035306));
#78136=CARTESIAN_POINT('Origin',(0.4,-1.84394625803399,15.4492861094852));
#78137=CARTESIAN_POINT('Origin',(0.400000000000001,-1.84394625804893,15.4492861094764));
#78138=CARTESIAN_POINT('Origin',(0.75,0.,0.));
#78139=CARTESIAN_POINT('Origin',(0.,3.93404948555832,14.6820725595938));
#78140=CARTESIAN_POINT('',(0.,3.93404948555832,14.6820725595938));
#78141=CARTESIAN_POINT('Origin',(1.27397318515336,16.5357324406311,8.32667268468867E-16));
#78142=CARTESIAN_POINT('',(1.27397318515336,16.8803613012335,0.203054053000301));
#78143=CARTESIAN_POINT('',(1.27397318515336,16.8803613012335,-0.203054053000298));
#78144=CARTESIAN_POINT('Origin',(1.27397318515336,16.5357324406311,8.32667268468867E-16));
#78145=CARTESIAN_POINT('',(0.975876659743317,16.802450384419,6.93889390390723E-16));
#78146=CARTESIAN_POINT('Origin',(1.27397318515336,16.5357324406311,8.32667268468867E-16));
#78147=CARTESIAN_POINT('Origin',(1.27397318515336,16.5357324406311,8.32667268468867E-16));
#78148=CARTESIAN_POINT('Origin',(0.,16.5357324406311,2.77555756156289E-16));
#78149=CARTESIAN_POINT('',(0.,16.8803613012335,0.2030540530003));
#78150=CARTESIAN_POINT('',(0.,16.8803613012335,-0.2030540530003));
#78151=CARTESIAN_POINT('Origin',(0.,17.,0.));
#78152=CARTESIAN_POINT('Ctrl Pts',(-6.07153216591882E-16,15.1775971465514,
3.09303168128218));
#78153=CARTESIAN_POINT('Ctrl Pts',(0.342254158915971,15.7598468593239,2.10482163507042));
#78154=CARTESIAN_POINT('Ctrl Pts',(0.778976516072333,16.3271297299077,1.14201372042963));
#78155=CARTESIAN_POINT('Ctrl Pts',(1.27397318515336,16.8803613012335,0.2030540530003));
#78156=CARTESIAN_POINT('',(0.,14.6820725595938,3.93404948555832));
#78157=CARTESIAN_POINT('Ctrl Pts',(0.975876659743317,16.802450384419,2.08166817117217E-16));
#78158=CARTESIAN_POINT('Ctrl Pts',(0.480879990662293,16.2492188130932,0.954104892637566));
#78159=CARTESIAN_POINT('Ctrl Pts',(0.0441576335059318,15.6806630308962,
1.9340418221227));
#78160=CARTESIAN_POINT('Ctrl Pts',(-0.29809652541004,15.094763561356,2.9409844446204));
#78161=CARTESIAN_POINT('Ctrl Pts',(1.04274635983407,16.8771871080498,0.0792866791192669));
#78162=CARTESIAN_POINT('Ctrl Pts',(0.549500375191472,16.3212686006415,1.02935818638529));
#78163=CARTESIAN_POINT('Ctrl Pts',(0.114335946070695,15.7506463874951,2.00456988736671));
#78164=CARTESIAN_POINT('Ctrl Pts',(-0.226532942966501,15.1635275167127,
3.00628506286562));
#78165=CARTESIAN_POINT('Ctrl Pts',(1.15757519551697,16.9071989300679,0.157504499520385));
#78166=CARTESIAN_POINT('Ctrl Pts',(0.663547764345894,16.3510761827228,1.10120348524803));
#78167=CARTESIAN_POINT('Ctrl Pts',(0.22765535797553,15.7807541837498,2.06945687194284));
#78168=CARTESIAN_POINT('Ctrl Pts',(-0.113842189164375,15.1948414649144,
3.06376415521458));
#78169=CARTESIAN_POINT('Ctrl Pts',(1.27397318515336,16.8803613012335,0.2030540530003));
#78170=CARTESIAN_POINT('Ctrl Pts',(0.778976516072333,16.3271297299077,1.14201372042963));
#78171=CARTESIAN_POINT('Ctrl Pts',(0.342254158915971,15.7598468593239,2.10482163507042));
#78172=CARTESIAN_POINT('Ctrl Pts',(-6.07153216591882E-16,15.1775971465514,
3.09303168128218));
#78173=CARTESIAN_POINT('',(0.10190347458996,15.71412433885,1.87555596859357));
#78174=CARTESIAN_POINT('Ctrl Pts',(0.975876659743317,16.802450384419,2.08166817117217E-16));
#78175=CARTESIAN_POINT('Ctrl Pts',(0.65714070715735,16.44621608447,0.614362784271561));
#78176=CARTESIAN_POINT('Ctrl Pts',(0.362566856291261,16.083627953311,1.23943622785986));
#78177=CARTESIAN_POINT('Ctrl Pts',(0.101818320067197,15.7141468216755,1.87553367897297));
#78178=CARTESIAN_POINT('Ctrl Pts',(0.10190347458996,15.71412433885,1.87555596859357));
#78179=CARTESIAN_POINT('Ctrl Pts',(0.101531729680471,15.7134655648902,1.87756967457526));
#78180=CARTESIAN_POINT('Ctrl Pts',(0.101161004946491,15.7128057829996,1.87958324464881));
#78181=CARTESIAN_POINT('Ctrl Pts',(0.0322254513574743,15.5895951744704,
2.25500838424547));
#78182=CARTESIAN_POINT('Ctrl Pts',(5.32975463135697E-16,15.4357465045314,
2.61362864336884));
#78183=CARTESIAN_POINT('Ctrl Pts',(3.46944695195361E-17,15.2868391646771,
2.89708947882623));
#78184=CARTESIAN_POINT('Ctrl Pts',(-0.29809652541004,15.094763561356,-2.9409844446204));
#78185=CARTESIAN_POINT('Ctrl Pts',(0.0441576335059358,15.6806630308962,
-1.9340418221227));
#78186=CARTESIAN_POINT('Ctrl Pts',(0.480879990662291,16.2492188130932,-0.954104892637568));
#78187=CARTESIAN_POINT('Ctrl Pts',(0.975876659743318,16.802450384419,2.77555756156289E-15));
#78188=CARTESIAN_POINT('Ctrl Pts',(-0.2265329429665,15.1635275167127,-3.00628506286562));
#78189=CARTESIAN_POINT('Ctrl Pts',(0.114335946070699,15.7506463874951,-2.00456988736671));
#78190=CARTESIAN_POINT('Ctrl Pts',(0.54950037519147,16.3212686006415,-1.02935818638529));
#78191=CARTESIAN_POINT('Ctrl Pts',(1.04274635983407,16.8771871080498,-0.079286679119264));
#78192=CARTESIAN_POINT('Ctrl Pts',(-0.113842189164374,15.1948414649144,
-3.06376415521458));
#78193=CARTESIAN_POINT('Ctrl Pts',(0.227655357975533,15.7807541837498,-2.06945687194284));
#78194=CARTESIAN_POINT('Ctrl Pts',(0.663547764345893,16.3510761827228,-1.10120348524803));
#78195=CARTESIAN_POINT('Ctrl Pts',(1.15757519551698,16.9071989300679,-0.157504499520383));
#78196=CARTESIAN_POINT('Ctrl Pts',(1.73472347597681E-17,15.1775971465514,
-3.09303168128219));
#78197=CARTESIAN_POINT('Ctrl Pts',(0.342254158915975,15.7598468593239,-2.10482163507042));
#78198=CARTESIAN_POINT('Ctrl Pts',(0.778976516072331,16.3271297299077,-1.14201372042963));
#78199=CARTESIAN_POINT('Ctrl Pts',(1.27397318515336,16.8803613012335,-0.203054053000297));
#78200=CARTESIAN_POINT('Ctrl Pts',(1.27397318515336,16.8803613012335,-0.203054053000297));
#78201=CARTESIAN_POINT('Ctrl Pts',(0.778976516072331,16.3271297299077,-1.14201372042963));
#78202=CARTESIAN_POINT('Ctrl Pts',(0.342254158915975,15.7598468593239,-2.10482163507042));
#78203=CARTESIAN_POINT('Ctrl Pts',(1.73472347597681E-17,15.1775971465514,
-3.09303168128219));
#78204=CARTESIAN_POINT('',(0.10190347458996,15.71412433885,-1.87555596859357));
#78205=CARTESIAN_POINT('Ctrl Pts',(-2.60208521396521E-17,15.2868391646771,
-2.89708947882622));
#78206=CARTESIAN_POINT('Ctrl Pts',(-2.60208521396521E-17,15.4357465045086,
-2.61362864341215));
#78207=CARTESIAN_POINT('Ctrl Pts',(0.0322254513462263,15.5895951744505,
-2.25500838430496));
#78208=CARTESIAN_POINT('Ctrl Pts',(0.101161004946562,15.7128057829998,-1.87958324464846));
#78209=CARTESIAN_POINT('Ctrl Pts',(0.10153172968041,15.7134655648901,-1.87756967457559));
#78210=CARTESIAN_POINT('Ctrl Pts',(0.10190347458996,15.71412433885,-1.87555596859357));
#78211=CARTESIAN_POINT('Ctrl Pts',(0.101818320067199,15.7141468216755,-1.87553367897297));
#78212=CARTESIAN_POINT('Ctrl Pts',(0.362566856291262,16.083627953311,-1.23943622785986));
#78213=CARTESIAN_POINT('Ctrl Pts',(0.65714070715735,16.44621608447,-0.614362784271561));
#78214=CARTESIAN_POINT('Ctrl Pts',(0.975876659743318,16.802450384419,2.77555756156289E-15));
#78215=CARTESIAN_POINT('Origin',(1.27397318515336,14.320364363769,8.26786622031553));
#78216=CARTESIAN_POINT('',(1.27397318515336,14.5172946854278,8.61603061885642));
#78217=CARTESIAN_POINT('',(1.27397318515336,14.7203487384281,8.26433068237711));
#78218=CARTESIAN_POINT('Origin',(1.27397318515336,14.320364363769,8.26786622031553));
#78219=CARTESIAN_POINT('',(0.975876659743319,14.5513488787345,8.4012251922095));
#78220=CARTESIAN_POINT('Origin',(1.27397318515336,14.320364363769,8.26786622031553));
#78221=CARTESIAN_POINT('Origin',(1.27397318515336,14.320364363769,8.26786622031553));
#78222=CARTESIAN_POINT('Origin',(0.,14.320364363769,8.26786622031553));
#78223=CARTESIAN_POINT('',(0.,14.5172946854278,8.61603061885642));
#78224=CARTESIAN_POINT('',(0.,14.7203487384281,8.26433068237712));
#78225=CARTESIAN_POINT('Origin',(0.,14.7224318643355,8.5));
#78226=CARTESIAN_POINT('Ctrl Pts',(1.73472347597681E-17,11.5976688566786,
10.2674425839762));
#78227=CARTESIAN_POINT('Ctrl Pts',(0.342255094986009,12.596019652888,9.70275089163238));
#78228=CARTESIAN_POINT('Ctrl Pts',(0.778977013899441,13.568703210786,9.15257721870111));
#78229=CARTESIAN_POINT('Ctrl Pts',(1.27397318515336,14.5172946854278,8.61603061885642));
#78230=CARTESIAN_POINT('',(0.4,10.7480230740355,10.7480230740355));
#78231=CARTESIAN_POINT('Origin',(0.4,10.0722782811866,11.1302408997889));
#78232=CARTESIAN_POINT('',(0.,10.7480230740355,10.7480230740355));
#78233=CARTESIAN_POINT('Ctrl Pts',(0.975876659743319,14.5513488787345,8.4012251922095));
#78234=CARTESIAN_POINT('Ctrl Pts',(0.480880488489401,13.5951847991044,8.95088792863941));
#78235=CARTESIAN_POINT('Ctrl Pts',(0.0441585695759698,12.6128343866363,
9.51525928157349));
#78236=CARTESIAN_POINT('Ctrl Pts',(-0.29809652541004,11.6019564859438,10.0943490218541));
#78237=CARTESIAN_POINT('Ctrl Pts',(1.04274635983407,14.5764294404348,8.50725783232391));
#78238=CARTESIAN_POINT('Ctrl Pts',(0.549500871257885,13.6199550988967,9.05208409138169));
#78239=CARTESIAN_POINT('Ctrl Pts',(0.114336878351999,12.6381777144107,9.61133007010324));
#78240=CARTESIAN_POINT('Ctrl Pts',(-0.2265329429665,11.6288575090247,10.1852829938157));
#78241=CARTESIAN_POINT('Ctrl Pts',(1.15757519551698,14.5633115305157,8.59000236282894));
#78242=CARTESIAN_POINT('Ctrl Pts',(0.663548261198221,13.6098465697466,9.12920774203302));
#78243=CARTESIAN_POINT('Ctrl Pts',(0.227656291976223,12.631808325544,9.68257776114536));
#78244=CARTESIAN_POINT('Ctrl Pts',(-0.113842189164374,11.6272366374857,
10.2507183220772));
#78245=CARTESIAN_POINT('Ctrl Pts',(1.27397318515336,14.5172946854278,8.61603061885642));
#78246=CARTESIAN_POINT('Ctrl Pts',(0.778977013899441,13.568703210786,9.15257721870111));
#78247=CARTESIAN_POINT('Ctrl Pts',(0.342255094986009,12.596019652888,9.70275089163238));
#78248=CARTESIAN_POINT('Ctrl Pts',(1.73472347597681E-17,11.5976688566786,
10.2674425839762));
#78249=CARTESIAN_POINT('',(0.101903474589961,12.6710528913746,9.48134128444654));
#78250=CARTESIAN_POINT('Ctrl Pts',(0.975876659743319,14.5513488787345,8.4012251922095));
#78251=CARTESIAN_POINT('Ctrl Pts',(0.6571407874074,13.9356596881592,8.75516173144116));
#78252=CARTESIAN_POINT('Ctrl Pts',(0.362567028519819,13.3091129212202,9.11519686904807));
#78253=CARTESIAN_POINT('Ctrl Pts',(0.101818266846041,12.6710835238972,9.48133321370127));
#78254=CARTESIAN_POINT('Ctrl Pts',(0.101903474589962,12.6710528913746,9.48134128444654));
#78255=CARTESIAN_POINT('Ctrl Pts',(0.101531854875395,12.6694760546196,9.482755341621));
#78256=CARTESIAN_POINT('Ctrl Pts',(0.101161254638804,12.6678984134239,9.48416877758682));
#78257=CARTESIAN_POINT('Ctrl Pts',(0.0322255749794838,12.3734824350501,
9.74769125268985));
#78258=CARTESIAN_POINT('Ctrl Pts',(3.3218792304595E-17,12.0609347982382,
9.98134172453387));
#78259=CARTESIAN_POINT('Ctrl Pts',(0.,11.7902463207642,10.1523726680387));
#78260=CARTESIAN_POINT('Ctrl Pts',(-0.29809652541004,14.5429409305642,5.00041453950186));
#78261=CARTESIAN_POINT('Ctrl Pts',(0.0441692435015672,14.5468735774003,
6.16544168438893));
#78262=CARTESIAN_POINT('Ctrl Pts',(0.480866735040972,14.5492886749403,7.29830079699084));
#78263=CARTESIAN_POINT('Ctrl Pts',(0.975876659743319,14.5513488787345,8.4012251922095));
#78264=CARTESIAN_POINT('Ctrl Pts',(-0.2265329429665,14.6351425718904,4.97824452289702));
#78265=CARTESIAN_POINT('Ctrl Pts',(0.114347509075003,14.642745099165,6.13935413362065));
#78266=CARTESIAN_POINT('Ctrl Pts',(0.549487166452103,14.6493121518488,7.26915448422417));
#78267=CARTESIAN_POINT('Ctrl Pts',(1.04274635983407,14.655716119554,8.36992927572593));
#78268=CARTESIAN_POINT('Ctrl Pts',(-0.113842189164374,14.6910007927003,
4.94412314283721));
#78269=CARTESIAN_POINT('Ctrl Pts',(0.227666942305269,14.7012627980738,6.09821401664757));
#78270=CARTESIAN_POINT('Ctrl Pts',(0.663534534680001,14.7110488345259,7.22183856636074));
#78271=CARTESIAN_POINT('Ctrl Pts',(1.15757519551698,14.7208160300361,8.31719656723893));
#78272=CARTESIAN_POINT('Ctrl Pts',(1.04083408558608E-16,14.6907005379608,
4.91015456257522));
#78273=CARTESIAN_POINT('Ctrl Pts',(0.342265768911606,14.7008389013655,6.05713332991757));
#78274=CARTESIAN_POINT('Ctrl Pts',(0.778963260451011,14.7107157192413,7.17452278817499));
#78275=CARTESIAN_POINT('Ctrl Pts',(1.27397318515336,14.7203487384281,8.26433068237711));
#78276=CARTESIAN_POINT('Ctrl Pts',(1.27397318515336,14.7203487384281,8.26433068237711));
#78277=CARTESIAN_POINT('Ctrl Pts',(0.778963260451011,14.7107157192413,7.17452278817499));
#78278=CARTESIAN_POINT('Ctrl Pts',(0.342265768911606,14.7008389013655,6.05713332991757));
#78279=CARTESIAN_POINT('Ctrl Pts',(1.04083408558608E-16,14.6907005379608,
4.91015456257522));
#78280=CARTESIAN_POINT('',(0.10190347458996,14.5466088599682,6.23278305440342));
#78281=CARTESIAN_POINT('Ctrl Pts',(-8.67361737988404E-17,14.6873357995904,
5.13446649663844));
#78282=CARTESIAN_POINT('Ctrl Pts',(-8.67361737988404E-17,14.674562895875,
5.45440508002074));
#78283=CARTESIAN_POINT('Ctrl Pts',(0.0322255776869445,14.6284894666425,
5.84190452909785));
#78284=CARTESIAN_POINT('Ctrl Pts',(0.101161260605365,14.5474802948742,6.22863748316639));
#78285=CARTESIAN_POINT('Ctrl Pts',(0.101531857865739,14.5470450475163,6.23071046180659));
#78286=CARTESIAN_POINT('Ctrl Pts',(0.10190347458996,14.5466088599682,6.23278305440342));
#78287=CARTESIAN_POINT('Ctrl Pts',(0.101816772550151,14.5466172059265,6.23281415542458));
#78288=CARTESIAN_POINT('Ctrl Pts',(0.362562998261092,14.5485485235528,6.96842719743842));
#78289=CARTESIAN_POINT('Ctrl Pts',(0.65713076867369,14.5500222760516,7.69103212012555));
#78290=CARTESIAN_POINT('Ctrl Pts',(0.975876659743319,14.5513488787345,8.4012251922095));
#78291=CARTESIAN_POINT('Origin',(1.27397318515336,8.26786622031554,14.320364363769));
#78292=CARTESIAN_POINT('',(1.27397318515336,8.26433068237712,14.7203487384281));
#78293=CARTESIAN_POINT('',(1.27397318515336,8.61603061885642,14.5172946854278));
#78294=CARTESIAN_POINT('Origin',(1.27397318515336,8.26786622031554,14.320364363769));
#78295=CARTESIAN_POINT('',(0.975876659743318,8.4012251922095,14.5513488787345));
#78296=CARTESIAN_POINT('Origin',(1.27397318515336,8.26786622031554,14.320364363769));
#78297=CARTESIAN_POINT('Origin',(1.27397318515336,8.26786622031554,14.320364363769));
#78298=CARTESIAN_POINT('Origin',(0.,8.26786622031554,14.320364363769));
#78299=CARTESIAN_POINT('',(0.,8.26433068237712,14.7203487384281));
#78300=CARTESIAN_POINT('',(0.,8.61603061885642,14.5172946854278));
#78301=CARTESIAN_POINT('Origin',(0.,8.5,14.7224318643355));
#78302=CARTESIAN_POINT('',(0.400000000002955,6.12420321413256,14.7014317448244));
#78303=CARTESIAN_POINT('Ctrl Pts',(0.400000000000002,6.12420321411613,14.7014317448242));
#78304=CARTESIAN_POINT('Ctrl Pts',(0.660836697158373,6.84944850421848,14.7078423258376));
#78305=CARTESIAN_POINT('Ctrl Pts',(0.955206208779907,7.56253714263826,14.7141454518953));
#78306=CARTESIAN_POINT('Ctrl Pts',(1.27397318515336,8.26433068237712,14.7203487384281));
#78307=CARTESIAN_POINT('',(0.4,4.18526992814786,14.6842931448515));
#78308=CARTESIAN_POINT('Ctrl Pts',(0.975876659743319,8.4012251922095,14.5513488787345));
#78309=CARTESIAN_POINT('Ctrl Pts',(0.657109683369867,7.69098514026756,14.5500221882957));
#78310=CARTESIAN_POINT('Ctrl Pts',(0.362740171748333,6.96849262263024,14.5485358134915));
#78311=CARTESIAN_POINT('Ctrl Pts',(0.101903474589963,6.23278305440343,14.5466088599682));
#78312=CARTESIAN_POINT('Ctrl Pts',(1.04274635983407,8.36992927572593,14.655716119554));
#78313=CARTESIAN_POINT('Ctrl Pts',(0.725106785764269,7.66107348426655,14.6515922155264));
#78314=CARTESIAN_POINT('Ctrl Pts',(0.431748041043183,6.94036445765127,14.6474504130738));
#78315=CARTESIAN_POINT('Ctrl Pts',(0.171922236290507,6.20674945042512,14.6429006199952));
#78316=CARTESIAN_POINT('Ctrl Pts',(1.15757519551698,8.31719656723893,14.7208160300361));
#78317=CARTESIAN_POINT('Ctrl Pts',(0.839432387056639,7.61182897648534,14.7145263392136));
#78318=CARTESIAN_POINT('Ctrl Pts',(0.545602236873283,6.89490956213576,14.7082901641236));
#78319=CARTESIAN_POINT('Ctrl Pts',(0.28532016266532,6.16544494773845,14.7017962883492));
#78320=CARTESIAN_POINT('Ctrl Pts',(1.27397318515336,8.26433068237712,14.7203487384281));
#78321=CARTESIAN_POINT('Ctrl Pts',(0.955206208779907,7.56253714263826,14.7141454518953));
#78322=CARTESIAN_POINT('Ctrl Pts',(0.660836697158373,6.84944850421848,14.7078423258376));
#78323=CARTESIAN_POINT('Ctrl Pts',(0.400000000000002,6.12420321411613,14.7014317448242));
#78324=CARTESIAN_POINT('',(0.101903474589964,6.23278305440343,14.5466088599682));
#78325=CARTESIAN_POINT('Ctrl Pts',(0.975876659743319,8.4012251922095,14.5513488787345));
#78326=CARTESIAN_POINT('Ctrl Pts',(0.657109683369867,7.69098514026756,14.5500221882957));
#78327=CARTESIAN_POINT('Ctrl Pts',(0.362740171748333,6.96849262263024,14.5485358134915));
#78328=CARTESIAN_POINT('Ctrl Pts',(0.101903474589963,6.23278305440343,14.5466088599682));
#78329=CARTESIAN_POINT('Origin',(0.400000000000003,6.12773875205455,14.3014473701651));
#78330=CARTESIAN_POINT('Ctrl Pts',(0.101903474589961,9.48134128444655,12.6710528913746));
#78331=CARTESIAN_POINT('Ctrl Pts',(0.362752890602842,9.11513743516542,13.3091906592268));
#78332=CARTESIAN_POINT('Ctrl Pts',(0.657115533348916,8.75518977451645,13.9356109059161));
#78333=CARTESIAN_POINT('Ctrl Pts',(0.975876659743319,8.4012251922095,14.5513488787345));
#78334=CARTESIAN_POINT('Ctrl Pts',(0.171922236290506,9.57774919679415,12.6966530089908));
#78335=CARTESIAN_POINT('Ctrl Pts',(0.431760710604808,9.21486423552519,13.3342882290803));
#78336=CARTESIAN_POINT('Ctrl Pts',(0.725112615053345,8.85810788352041,13.960491669232));
#78337=CARTESIAN_POINT('Ctrl Pts',(1.04274635983407,8.50725783232391,14.5764294404348));
#78338=CARTESIAN_POINT('Ctrl Pts',(0.285320162665318,9.64940659310495,12.6903300945505));
#78339=CARTESIAN_POINT('Ctrl Pts',(0.545614928683405,9.29028063653872,13.3253428824943));
#78340=CARTESIAN_POINT('Ctrl Pts',(0.839438225581022,8.93723275371785,13.9493117007747));
#78341=CARTESIAN_POINT('Ctrl Pts',(1.15757519551698,8.59000236282894,14.5633115305157));
#78342=CARTESIAN_POINT('Ctrl Pts',(0.400000000000001,9.6697117559627,12.654431433775));
#78343=CARTESIAN_POINT('Ctrl Pts',(0.660849416012883,9.31262342551825,13.2857483521037));
#78344=CARTESIAN_POINT('Ctrl Pts',(0.955212058758955,8.96154884396982,13.9064332192088));
#78345=CARTESIAN_POINT('Ctrl Pts',(1.27397318515336,8.61603061885642,14.5172946854278));
#78346=CARTESIAN_POINT('',(0.400000000002489,9.66971175595589,12.654431433787));
#78347=CARTESIAN_POINT('Ctrl Pts',(1.27397318515336,8.61603061885642,14.5172946854278));
#78348=CARTESIAN_POINT('Ctrl Pts',(0.955212058758955,8.96154884396982,13.9064332192088));
#78349=CARTESIAN_POINT('Ctrl Pts',(0.660849416012883,9.31262342551825,13.2857483521037));
#78350=CARTESIAN_POINT('Ctrl Pts',(0.400000000000001,9.6697117559627,12.654431433775));
#78351=CARTESIAN_POINT('',(0.101903474589964,9.48134128444654,12.6710528913746));
#78352=CARTESIAN_POINT('Origin',(0.400000000000003,9.32154735742182,12.4575011121161));
#78353=CARTESIAN_POINT('Ctrl Pts',(0.101903474589961,9.48134128444655,12.6710528913746));
#78354=CARTESIAN_POINT('Ctrl Pts',(0.362752890602842,9.11513743516542,13.3091906592268));
#78355=CARTESIAN_POINT('Ctrl Pts',(0.657115533348916,8.75518977451645,13.9356109059161));
#78356=CARTESIAN_POINT('Ctrl Pts',(0.975876659743319,8.4012251922095,14.5513488787345));
#78357=CARTESIAN_POINT('Origin',(0.4,11.4001830744621,8.78256193508806));
#78358=CARTESIAN_POINT('Origin',(0.4,9.32154735741501,12.4575011121282));
#78359=CARTESIAN_POINT('',(0.4,11.748347473003,8.97949225674692));
#78360=CARTESIAN_POINT('Origin',(0.4,0.,0.));
#78361=CARTESIAN_POINT('Origin',(0.4,6.12773875205455,14.3014473701651));
#78362=CARTESIAN_POINT('Origin',(0.101903474589959,-1.11022302462516E-15,
0.));
#78363=CARTESIAN_POINT('Origin',(0.4,9.32154735742181,12.4575011121161));
#78364=CARTESIAN_POINT('Origin',(0.400000000000003,9.32154735742182,12.4575011121161));
#78365=CARTESIAN_POINT('Origin',(0.4,4.18880546608628,14.2843087701924));
#78366=CARTESIAN_POINT('Origin',(0.4,6.12773875207098,14.3014473701652));
#78367=CARTESIAN_POINT('Origin',(0.400000000000003,6.12773875205455,14.3014473701651));
#78368=CARTESIAN_POINT('Origin',(0.75,0.,0.));
#78369=CARTESIAN_POINT('Origin',(0.,10.7480230740355,10.7480230740355));
#78370=CARTESIAN_POINT('Origin',(0.4,0.,0.));
#78371=CARTESIAN_POINT('Origin',(0.101903474589961,0.,0.));
#78372=CARTESIAN_POINT('Origin',(0.,14.6820725595938,3.93404948555832));
#78373=CARTESIAN_POINT('Origin',(0.75,0.,0.));
#78374=CARTESIAN_POINT('Origin',(0.4,0.,0.));
#78375=CARTESIAN_POINT('Origin',(0.10190347458996,0.,-9.69041998728974E-16));
#78376=CARTESIAN_POINT('Origin',(0.,14.6820725595938,-3.93404948555831));
#78377=CARTESIAN_POINT('Origin',(0.75,0.,0.));
#78378=CARTESIAN_POINT('Origin',(0.,-10.7480230740355,10.7480230740355));
#78379=CARTESIAN_POINT('Origin',(0.,-3.12284933782575E-15,-17.));
#78380=CARTESIAN_POINT('Origin',(0.,-8.50000000000001,-14.7224318643355));
#90340=UNCERTAINTY_MEASURE_WITH_UNIT(LENGTH_MEASURE(0.01),#90375,
'DISTANCE_ACCURACY_VALUE',
'Maximum model space distance between geometric entities at asserted c
onnectivities');
#90355=UNCERTAINTY_MEASURE_WITH_UNIT(LENGTH_MEASURE(0.01),#90375,
'DISTANCE_ACCURACY_VALUE',
'Maximum model space distance between geometric entities at asserted c
onnectivities');
#90359=(
GEOMETRIC_REPRESENTATION_CONTEXT(3)
GLOBAL_UNCERTAINTY_ASSIGNED_CONTEXT((#90340))
GLOBAL_UNIT_ASSIGNED_CONTEXT((#90375,#90377,#90378))
REPRESENTATION_CONTEXT('','3D')
);
#90374=(
GEOMETRIC_REPRESENTATION_CONTEXT(3)
GLOBAL_UNCERTAINTY_ASSIGNED_CONTEXT((#90355))
GLOBAL_UNIT_ASSIGNED_CONTEXT((#90375,#90377,#90378))
REPRESENTATION_CONTEXT('','3D')
);
#90375=(
LENGTH_UNIT()
NAMED_UNIT(*)
SI_UNIT(.MILLI.,.METRE.)
);
#90377=(
NAMED_UNIT(*)
PLANE_ANGLE_UNIT()
SI_UNIT($,.RADIAN.)
);
#90378=(
NAMED_UNIT(*)
SI_UNIT($,.STERADIAN.)
SOLID_ANGLE_UNIT()
);
#90382=SHAPE_DEFINITION_REPRESENTATION(#90400,#90443);
#90400=PRODUCT_DEFINITION_SHAPE('',$,#90462);
#90443=SHAPE_REPRESENTATION('',(#42998),#90359);
#90458=PRODUCT_DEFINITION_CONTEXT('part definition',#90514,'design');
#90462=PRODUCT_DEFINITION('2026-10-11-12-53-09-092',
'03_Axle_Nut_12-Point_Flange_M22x1.5',#90480,#90458);
#90480=PRODUCT_DEFINITION_FORMATION('',$,#90519);
#90514=APPLICATION_CONTEXT(
'Core Data for Automotive Mechanical Design Process');
#90515=PRODUCT_CONTEXT('part definition',#90514,'mechanical');
#90519=PRODUCT('2026-10-11-12-53-09-092',
'03_Axle_Nut_12-Point_Flange_M22x1.5',$,(#90515));
#90688=COLOUR_RGB('Black',0.12,0.14,0.17);
#90689=FILL_AREA_STYLE_COLOUR('',#90688);
#90690=FILL_AREA_STYLE('',(#90689));
#90691=SURFACE_STYLE_FILL_AREA(#90690);
#90692=SURFACE_SIDE_STYLE('',(#90691));
#90693=SURFACE_STYLE_USAGE(.BOTH.,#90692);
#90694=PRESENTATION_STYLE_ASSIGNMENT((#90693));
ENDSEC;
END-ISO-10303-21;
